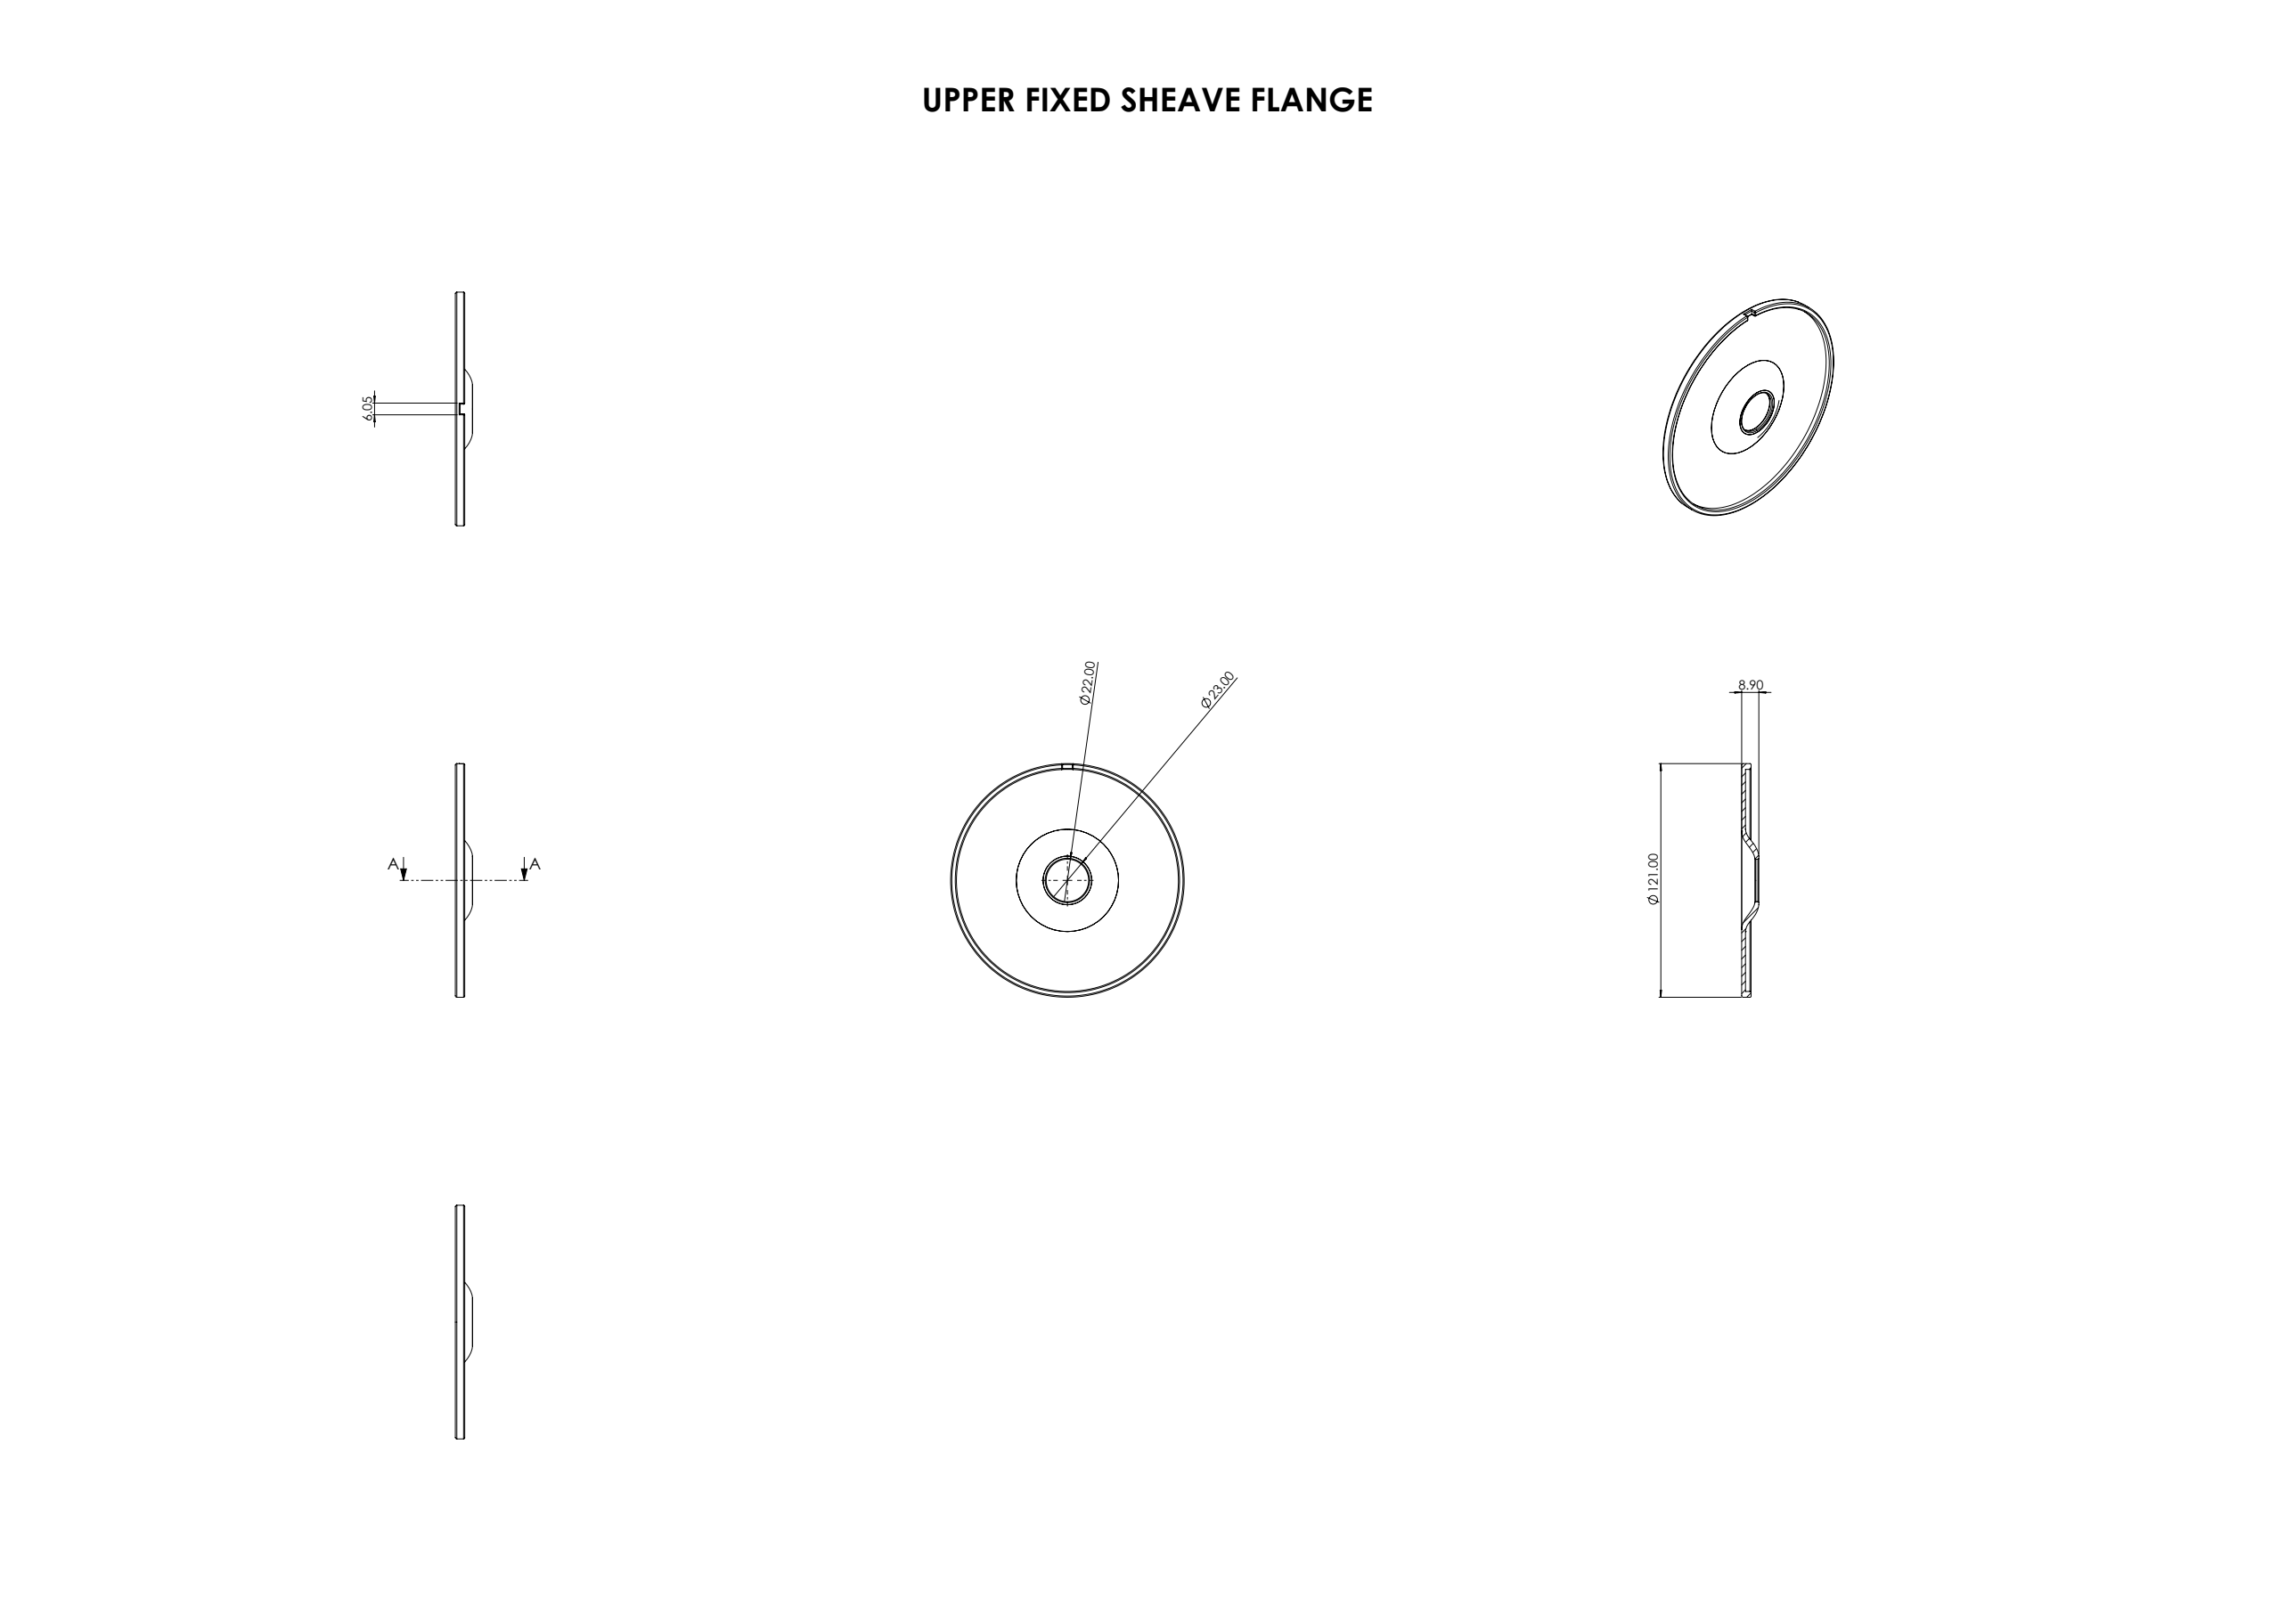
ISO-10303-21;
HEADER;
/* Generated by software containing ST-Developer
 * from STEP Tools, Inc. (www.steptools.com) 
 */

FILE_DESCRIPTION(
/* description */ (''),
/* implementation_level */ '2;1');

FILE_NAME(
/* name */ '01_Upper_Fixed_Sheave_Flange.step',
/* time_stamp */ '2026-10-24T13:41:11-07:00',
/* author */ (''),
/* organization */ (''),
/* preprocessor_version */ 'ST-DEVELOPER v20.2',
/* originating_system */ 'Autodesk Translation Framework v15.15.0.0',
/* authorisation */ '');

FILE_SCHEMA (('AUTOMOTIVE_DESIGN { 1 0 10303 214 3 1 1 }'));
ENDSEC;

DATA;
#10=MECHANICAL_DESIGN_GEOMETRIC_PRESENTATION_REPRESENTATION('',(#121),#12813);
#101=SHAPE_REPRESENTATION_RELATIONSHIP('SRR','None',#12854,#111);
#111=ADVANCED_BREP_SHAPE_REPRESENTATION('',(#131),#12803);
#121=STYLED_ITEM('',(#12960),#131);
#131=MANIFOLD_SOLID_BREP('Body1',#4384);
#141=FACE_BOUND('',#599,.T.);
#142=FACE_BOUND('',#604,.T.);
#143=FACE_BOUND('',#607,.T.);
#169=PLANE('',#4514);
#170=PLANE('',#4517);
#171=PLANE('',#4521);
#172=PLANE('',#4531);
#173=PLANE('',#4540);
#174=PLANE('',#4544);
#175=PLANE('',#4551);
#258=TOROIDAL_SURFACE('',#4511,11.5,0.5);
#259=TOROIDAL_SURFACE('',#4541,60.,0.5);
#260=TOROIDAL_SURFACE('',#4546,58.,0.5);
#261=TOROIDAL_SURFACE('',#4549,58.1,0.6);
#262=TOROIDAL_SURFACE('',#4558,59.9,0.6);
#263=TOROIDAL_SURFACE('',#4559,59.7,0.8);
#290=(
BOUNDED_CURVE()
B_SPLINE_CURVE(5,(#6647,#6648,#6649,#6650,#6651,#6652,#6653,#6654,#6655,
#6656,#6657,#6658,#6659,#6660,#6661,#6662,#6663,#6664,#6665,#6666,#6667,
#6668,#6669,#6670,#6671,#6672,#6673,#6674,#6675,#6676),.UNSPECIFIED.,.F.,
 .F.)
B_SPLINE_CURVE_WITH_KNOTS((6,1,1,1,1,1,1,1,1,1,1,1,1,1,1,1,1,1,1,1,1,1,
1,1,1,6),(8.37815962158244E-5,0.04,0.08,0.12,0.16,0.2,0.24,0.28,0.32,0.36,
0.4,0.44,0.48,0.52,0.56,0.6,0.64,0.68,0.72,0.76,0.8,0.84,0.88,0.92,0.96,
0.969915757295795),.UNSPECIFIED.)
CURVE()
GEOMETRIC_REPRESENTATION_ITEM()
RATIONAL_B_SPLINE_CURVE((1.,1.,1.,1.,1.,1.,1.,1.,1.,1.,1.,1.,1.,1.,1.,1.,
1.,1.,1.,1.,1.,1.,1.,1.,1.,1.,1.,1.,1.,1.))
REPRESENTATION_ITEM('')
);
#291=(
BOUNDED_CURVE()
B_SPLINE_CURVE(5,(#7077,#7078,#7079,#7080,#7081,#7082,#7083,#7084,#7085,
#7086,#7087,#7088,#7089,#7090,#7091,#7092,#7093,#7094,#7095,#7096,#7097,
#7098,#7099,#7100,#7101,#7102,#7103,#7104,#7105,#7106),.UNSPECIFIED.,.F.,
 .F.)
B_SPLINE_CURVE_WITH_KNOTS((6,1,1,1,1,1,1,1,1,1,1,1,1,1,1,1,1,1,1,1,1,1,
1,1,1,6),(0.00142562377953934,0.04,0.08,0.12,0.16,0.2,0.24,0.28,0.32,0.36,
0.4,0.44,0.48,0.52,0.56,0.6,0.64,0.68,0.72,0.76,0.8,0.84,0.88,0.92,0.96,
0.999682925140619),.UNSPECIFIED.)
CURVE()
GEOMETRIC_REPRESENTATION_ITEM()
RATIONAL_B_SPLINE_CURVE((1.,1.,1.,1.,1.,1.,1.,1.,1.,1.,1.,1.,1.,1.,1.,1.,
1.,1.,1.,1.,1.,1.,1.,1.,1.,1.,1.,1.,1.,1.))
REPRESENTATION_ITEM('')
);
#294=(
BOUNDED_SURFACE()
B_SPLINE_SURFACE(5,2,((#6376,#6377,#6378,#6379,#6380,#6381,#6382,#6383,
#6384),(#6385,#6386,#6387,#6388,#6389,#6390,#6391,#6392,#6393),(#6394,#6395,
#6396,#6397,#6398,#6399,#6400,#6401,#6402),(#6403,#6404,#6405,#6406,#6407,
#6408,#6409,#6410,#6411),(#6412,#6413,#6414,#6415,#6416,#6417,#6418,#6419,
#6420),(#6421,#6422,#6423,#6424,#6425,#6426,#6427,#6428,#6429),(#6430,#6431,
#6432,#6433,#6434,#6435,#6436,#6437,#6438),(#6439,#6440,#6441,#6442,#6443,
#6444,#6445,#6446,#6447),(#6448,#6449,#6450,#6451,#6452,#6453,#6454,#6455,
#6456),(#6457,#6458,#6459,#6460,#6461,#6462,#6463,#6464,#6465),(#6466,#6467,
#6468,#6469,#6470,#6471,#6472,#6473,#6474),(#6475,#6476,#6477,#6478,#6479,
#6480,#6481,#6482,#6483),(#6484,#6485,#6486,#6487,#6488,#6489,#6490,#6491,
#6492),(#6493,#6494,#6495,#6496,#6497,#6498,#6499,#6500,#6501),(#6502,#6503,
#6504,#6505,#6506,#6507,#6508,#6509,#6510),(#6511,#6512,#6513,#6514,#6515,
#6516,#6517,#6518,#6519),(#6520,#6521,#6522,#6523,#6524,#6525,#6526,#6527,
#6528),(#6529,#6530,#6531,#6532,#6533,#6534,#6535,#6536,#6537),(#6538,#6539,
#6540,#6541,#6542,#6543,#6544,#6545,#6546),(#6547,#6548,#6549,#6550,#6551,
#6552,#6553,#6554,#6555),(#6556,#6557,#6558,#6559,#6560,#6561,#6562,#6563,
#6564),(#6565,#6566,#6567,#6568,#6569,#6570,#6571,#6572,#6573),(#6574,#6575,
#6576,#6577,#6578,#6579,#6580,#6581,#6582),(#6583,#6584,#6585,#6586,#6587,
#6588,#6589,#6590,#6591),(#6592,#6593,#6594,#6595,#6596,#6597,#6598,#6599,
#6600),(#6601,#6602,#6603,#6604,#6605,#6606,#6607,#6608,#6609),(#6610,#6611,
#6612,#6613,#6614,#6615,#6616,#6617,#6618),(#6619,#6620,#6621,#6622,#6623,
#6624,#6625,#6626,#6627),(#6628,#6629,#6630,#6631,#6632,#6633,#6634,#6635,
#6636),(#6637,#6638,#6639,#6640,#6641,#6642,#6643,#6644,#6645)),
 .UNSPECIFIED.,.F.,.T.,.F.)
B_SPLINE_SURFACE_WITH_KNOTS((6,1,1,1,1,1,1,1,1,1,1,1,1,1,1,1,1,1,1,1,1,
1,1,1,1,6),(3,2,2,2,3),(0.,0.04,0.08,0.12,0.16,0.2,0.24,0.28,0.32,0.36,
0.4,0.44,0.48,0.52,0.56,0.6,0.64,0.68,0.72,0.76,0.8,0.84,0.88,0.92,0.96,
1.),(0.,1.5707963267949,3.14159265358979,4.71238898038469,6.28318530717959),
 .UNSPECIFIED.)
GEOMETRIC_REPRESENTATION_ITEM()
RATIONAL_B_SPLINE_SURFACE(((1.,0.707106781186548,1.,0.707106781186548,1.,
0.707106781186548,1.,0.707106781186548,1.),(1.,0.707106781186548,1.,0.707106781186548,
1.,0.707106781186548,1.,0.707106781186548,1.),(1.,0.707106781186548,1.,
0.707106781186548,1.,0.707106781186548,1.,0.707106781186548,1.),(1.,0.707106781186548,
1.,0.707106781186548,1.,0.707106781186548,1.,0.707106781186548,1.),(1.,
0.707106781186548,1.,0.707106781186548,1.,0.707106781186548,1.,0.707106781186548,
1.),(1.,0.707106781186548,1.,0.707106781186548,1.,0.707106781186548,1.,
0.707106781186548,1.),(1.,0.707106781186548,1.,0.707106781186548,1.,0.707106781186548,
1.,0.707106781186548,1.),(1.,0.707106781186548,1.,0.707106781186548,1.,
0.707106781186548,1.,0.707106781186548,1.),(1.,0.707106781186548,1.,0.707106781186548,
1.,0.707106781186548,1.,0.707106781186548,1.),(1.,0.707106781186548,1.,
0.707106781186548,1.,0.707106781186548,1.,0.707106781186548,1.),(1.,0.707106781186548,
1.,0.707106781186548,1.,0.707106781186548,1.,0.707106781186548,1.),(1.,
0.707106781186548,1.,0.707106781186548,1.,0.707106781186548,1.,0.707106781186548,
1.),(1.,0.707106781186548,1.,0.707106781186548,1.,0.707106781186548,1.,
0.707106781186548,1.),(1.,0.707106781186548,1.,0.707106781186548,1.,0.707106781186548,
1.,0.707106781186548,1.),(1.,0.707106781186548,1.,0.707106781186548,1.,
0.707106781186548,1.,0.707106781186548,1.),(1.,0.707106781186548,1.,0.707106781186548,
1.,0.707106781186548,1.,0.707106781186548,1.),(1.,0.707106781186548,1.,
0.707106781186548,1.,0.707106781186548,1.,0.707106781186548,1.),(1.,0.707106781186548,
1.,0.707106781186548,1.,0.707106781186548,1.,0.707106781186548,1.),(1.,
0.707106781186548,1.,0.707106781186548,1.,0.707106781186548,1.,0.707106781186548,
1.),(1.,0.707106781186548,1.,0.707106781186548,1.,0.707106781186548,1.,
0.707106781186548,1.),(1.,0.707106781186548,1.,0.707106781186548,1.,0.707106781186548,
1.,0.707106781186548,1.),(1.,0.707106781186548,1.,0.707106781186548,1.,
0.707106781186548,1.,0.707106781186548,1.),(1.,0.707106781186548,1.,0.707106781186548,
1.,0.707106781186548,1.,0.707106781186548,1.),(1.,0.707106781186548,1.,
0.707106781186548,1.,0.707106781186548,1.,0.707106781186548,1.),(1.,0.707106781186548,
1.,0.707106781186548,1.,0.707106781186548,1.,0.707106781186548,1.),(1.,
0.707106781186548,1.,0.707106781186548,1.,0.707106781186548,1.,0.707106781186548,
1.),(1.,0.707106781186548,1.,0.707106781186548,1.,0.707106781186548,1.,
0.707106781186548,1.),(1.,0.707106781186548,1.,0.707106781186548,1.,0.707106781186548,
1.,0.707106781186548,1.),(1.,0.707106781186548,1.,0.707106781186548,1.,
0.707106781186548,1.,0.707106781186548,1.),(1.,0.707106781186548,1.,0.707106781186548,
1.,0.707106781186548,1.,0.707106781186548,1.)))
REPRESENTATION_ITEM('')
SURFACE()
);
#295=(
BOUNDED_SURFACE()
B_SPLINE_SURFACE(5,2,((#6806,#6807,#6808,#6809,#6810,#6811,#6812,#6813,
#6814),(#6815,#6816,#6817,#6818,#6819,#6820,#6821,#6822,#6823),(#6824,#6825,
#6826,#6827,#6828,#6829,#6830,#6831,#6832),(#6833,#6834,#6835,#6836,#6837,
#6838,#6839,#6840,#6841),(#6842,#6843,#6844,#6845,#6846,#6847,#6848,#6849,
#6850),(#6851,#6852,#6853,#6854,#6855,#6856,#6857,#6858,#6859),(#6860,#6861,
#6862,#6863,#6864,#6865,#6866,#6867,#6868),(#6869,#6870,#6871,#6872,#6873,
#6874,#6875,#6876,#6877),(#6878,#6879,#6880,#6881,#6882,#6883,#6884,#6885,
#6886),(#6887,#6888,#6889,#6890,#6891,#6892,#6893,#6894,#6895),(#6896,#6897,
#6898,#6899,#6900,#6901,#6902,#6903,#6904),(#6905,#6906,#6907,#6908,#6909,
#6910,#6911,#6912,#6913),(#6914,#6915,#6916,#6917,#6918,#6919,#6920,#6921,
#6922),(#6923,#6924,#6925,#6926,#6927,#6928,#6929,#6930,#6931),(#6932,#6933,
#6934,#6935,#6936,#6937,#6938,#6939,#6940),(#6941,#6942,#6943,#6944,#6945,
#6946,#6947,#6948,#6949),(#6950,#6951,#6952,#6953,#6954,#6955,#6956,#6957,
#6958),(#6959,#6960,#6961,#6962,#6963,#6964,#6965,#6966,#6967),(#6968,#6969,
#6970,#6971,#6972,#6973,#6974,#6975,#6976),(#6977,#6978,#6979,#6980,#6981,
#6982,#6983,#6984,#6985),(#6986,#6987,#6988,#6989,#6990,#6991,#6992,#6993,
#6994),(#6995,#6996,#6997,#6998,#6999,#7000,#7001,#7002,#7003),(#7004,#7005,
#7006,#7007,#7008,#7009,#7010,#7011,#7012),(#7013,#7014,#7015,#7016,#7017,
#7018,#7019,#7020,#7021),(#7022,#7023,#7024,#7025,#7026,#7027,#7028,#7029,
#7030),(#7031,#7032,#7033,#7034,#7035,#7036,#7037,#7038,#7039),(#7040,#7041,
#7042,#7043,#7044,#7045,#7046,#7047,#7048),(#7049,#7050,#7051,#7052,#7053,
#7054,#7055,#7056,#7057),(#7058,#7059,#7060,#7061,#7062,#7063,#7064,#7065,
#7066),(#7067,#7068,#7069,#7070,#7071,#7072,#7073,#7074,#7075)),
 .UNSPECIFIED.,.F.,.T.,.F.)
B_SPLINE_SURFACE_WITH_KNOTS((6,1,1,1,1,1,1,1,1,1,1,1,1,1,1,1,1,1,1,1,1,
1,1,1,1,6),(3,2,2,2,3),(0.,0.04,0.08,0.12,0.16,0.2,0.24,0.28,0.32,0.36,
0.4,0.44,0.48,0.52,0.56,0.6,0.64,0.68,0.72,0.76,0.8,0.84,0.88,0.92,0.96,
1.),(0.,1.5707963267949,3.14159265358979,4.71238898038469,6.28318530717959),
 .UNSPECIFIED.)
GEOMETRIC_REPRESENTATION_ITEM()
RATIONAL_B_SPLINE_SURFACE(((1.,0.707106781186548,1.,0.707106781186548,1.,
0.707106781186548,1.,0.707106781186548,1.),(1.,0.707106781186548,1.,0.707106781186548,
1.,0.707106781186548,1.,0.707106781186548,1.),(1.,0.707106781186548,1.,
0.707106781186548,1.,0.707106781186548,1.,0.707106781186548,1.),(1.,0.707106781186548,
1.,0.707106781186548,1.,0.707106781186548,1.,0.707106781186548,1.),(1.,
0.707106781186548,1.,0.707106781186548,1.,0.707106781186548,1.,0.707106781186548,
1.),(1.,0.707106781186548,1.,0.707106781186548,1.,0.707106781186548,1.,
0.707106781186548,1.),(1.,0.707106781186548,1.,0.707106781186548,1.,0.707106781186548,
1.,0.707106781186548,1.),(1.,0.707106781186548,1.,0.707106781186548,1.,
0.707106781186548,1.,0.707106781186548,1.),(1.,0.707106781186548,1.,0.707106781186548,
1.,0.707106781186548,1.,0.707106781186548,1.),(1.,0.707106781186548,1.,
0.707106781186548,1.,0.707106781186548,1.,0.707106781186548,1.),(1.,0.707106781186548,
1.,0.707106781186548,1.,0.707106781186548,1.,0.707106781186548,1.),(1.,
0.707106781186548,1.,0.707106781186548,1.,0.707106781186548,1.,0.707106781186548,
1.),(1.,0.707106781186548,1.,0.707106781186548,1.,0.707106781186548,1.,
0.707106781186548,1.),(1.,0.707106781186548,1.,0.707106781186548,1.,0.707106781186548,
1.,0.707106781186548,1.),(1.,0.707106781186548,1.,0.707106781186548,1.,
0.707106781186548,1.,0.707106781186548,1.),(1.,0.707106781186548,1.,0.707106781186548,
1.,0.707106781186548,1.,0.707106781186548,1.),(1.,0.707106781186548,1.,
0.707106781186548,1.,0.707106781186548,1.,0.707106781186548,1.),(1.,0.707106781186548,
1.,0.707106781186548,1.,0.707106781186548,1.,0.707106781186548,1.),(1.,
0.707106781186548,1.,0.707106781186548,1.,0.707106781186548,1.,0.707106781186548,
1.),(1.,0.707106781186548,1.,0.707106781186548,1.,0.707106781186548,1.,
0.707106781186548,1.),(1.,0.707106781186548,1.,0.707106781186548,1.,0.707106781186548,
1.,0.707106781186548,1.),(1.,0.707106781186548,1.,0.707106781186548,1.,
0.707106781186548,1.,0.707106781186548,1.),(1.,0.707106781186548,1.,0.707106781186548,
1.,0.707106781186548,1.,0.707106781186548,1.),(1.,0.707106781186548,1.,
0.707106781186548,1.,0.707106781186548,1.,0.707106781186548,1.),(1.,0.707106781186548,
1.,0.707106781186548,1.,0.707106781186548,1.,0.707106781186548,1.),(1.,
0.707106781186548,1.,0.707106781186548,1.,0.707106781186548,1.,0.707106781186548,
1.),(1.,0.707106781186548,1.,0.707106781186548,1.,0.707106781186548,1.,
0.707106781186548,1.),(1.,0.707106781186548,1.,0.707106781186548,1.,0.707106781186548,
1.,0.707106781186548,1.),(1.,0.707106781186548,1.,0.707106781186548,1.,
0.707106781186548,1.,0.707106781186548,1.),(1.,0.707106781186548,1.,0.707106781186548,
1.,0.707106781186548,1.,0.707106781186548,1.)))
REPRESENTATION_ITEM('')
SURFACE()
);
#298=B_SPLINE_SURFACE_WITH_KNOTS('',3,3,((#6289,#6290,#6291,#6292,#6293,
#6294,#6295,#6296,#6297,#6298,#6299,#6300,#6301,#6302,#6303,#6304,#6305),
(#6306,#6307,#6308,#6309,#6310,#6311,#6312,#6313,#6314,#6315,#6316,#6317,
#6318,#6319,#6320,#6321,#6322),(#6323,#6324,#6325,#6326,#6327,#6328,#6329,
#6330,#6331,#6332,#6333,#6334,#6335,#6336,#6337,#6338,#6339),(#6340,#6341,
#6342,#6343,#6344,#6345,#6346,#6347,#6348,#6349,#6350,#6351,#6352,#6353,
#6354,#6355,#6356)),.UNSPECIFIED.,.F.,.T.,.F.,(4,4),(4,1,1,1,1,1,1,1,1,
1,1,1,1,1,4),(0.316273000492814,1.),(1.5707963267949,2.01959527730772,2.46839422782055,
2.91719317833338,3.36599212884621,3.96439072952998,4.26359002987186,4.56278933021375,
5.16118793089752,5.4603872312394,6.05878583192317,6.35798513226506,6.95638373294883,
7.40518268346166,7.85398163397448),.UNSPECIFIED.);
#299=B_SPLINE_SURFACE_WITH_KNOTS('',3,3,((#6719,#6720,#6721,#6722,#6723,
#6724,#6725,#6726,#6727,#6728,#6729,#6730,#6731,#6732,#6733,#6734,#6735),
(#6736,#6737,#6738,#6739,#6740,#6741,#6742,#6743,#6744,#6745,#6746,#6747,
#6748,#6749,#6750,#6751,#6752),(#6753,#6754,#6755,#6756,#6757,#6758,#6759,
#6760,#6761,#6762,#6763,#6764,#6765,#6766,#6767,#6768,#6769),(#6770,#6771,
#6772,#6773,#6774,#6775,#6776,#6777,#6778,#6779,#6780,#6781,#6782,#6783,
#6784,#6785,#6786)),.UNSPECIFIED.,.F.,.T.,.F.,(4,4),(4,1,1,1,1,1,1,1,1,
1,1,1,1,1,4),(0.,1.),(1.5707963267949,2.01959527730772,2.46839422782055,
2.91719317833338,3.36599212884621,3.66519142918809,4.26359002987186,4.56278933021375,
5.16118793089752,5.4603872312394,6.05878583192317,6.35798513226506,6.95638373294883,
7.40518268346166,7.85398163397448),.UNSPECIFIED.);
#300=B_SPLINE_SURFACE_WITH_KNOTS('',3,3,((#7126,#7127,#7128,#7129,#7130,
#7131,#7132,#7133,#7134,#7135,#7136,#7137,#7138,#7139,#7140,#7141,#7142,
#7143,#7144),(#7145,#7146,#7147,#7148,#7149,#7150,#7151,#7152,#7153,#7154,
#7155,#7156,#7157,#7158,#7159,#7160,#7161,#7162,#7163),(#7164,#7165,#7166,
#7167,#7168,#7169,#7170,#7171,#7172,#7173,#7174,#7175,#7176,#7177,#7178,
#7179,#7180,#7181,#7182),(#7183,#7184,#7185,#7186,#7187,#7188,#7189,#7190,
#7191,#7192,#7193,#7194,#7195,#7196,#7197,#7198,#7199,#7200,#7201)),
 .UNSPECIFIED.,.F.,.T.,.F.,(4,4),(4,1,1,1,1,1,1,1,1,1,1,1,1,1,1,1,4),(0.,
1.),(1.5707963267949,2.01959527730772,2.46839422782055,2.91719317833338,
3.36599212884621,3.66519142918809,3.96439072952998,4.26359002987186,4.56278933021375,
5.16118793089752,5.4603872312394,5.75958653158129,6.05878583192317,6.35798513226506,
6.95638373294883,7.40518268346166,7.85398163397448),.UNSPECIFIED.);
#301=B_SPLINE_SURFACE_WITH_KNOTS('',3,3,((#7228,#7229,#7230,#7231,#7232,
#7233,#7234,#7235,#7236,#7237,#7238,#7239,#7240,#7241,#7242,#7243,#7244,
#7245,#7246),(#7247,#7248,#7249,#7250,#7251,#7252,#7253,#7254,#7255,#7256,
#7257,#7258,#7259,#7260,#7261,#7262,#7263,#7264,#7265),(#7266,#7267,#7268,
#7269,#7270,#7271,#7272,#7273,#7274,#7275,#7276,#7277,#7278,#7279,#7280,
#7281,#7282,#7283,#7284),(#7285,#7286,#7287,#7288,#7289,#7290,#7291,#7292,
#7293,#7294,#7295,#7296,#7297,#7298,#7299,#7300,#7301,#7302,#7303)),
 .UNSPECIFIED.,.F.,.T.,.F.,(4,4),(4,1,1,1,1,1,1,1,1,1,1,1,1,1,1,1,4),(0.,
1.),(1.5707963267949,2.01959527730772,2.46839422782055,2.91719317833338,
3.36599212884621,3.66519142918809,3.96439072952998,4.26359002987186,4.56278933021375,
5.16118793089752,5.4603872312394,5.75958653158129,6.05878583192317,6.35798513226506,
6.95638373294883,7.40518268346166,7.85398163397448),.UNSPECIFIED.);
#302=B_SPLINE_SURFACE_WITH_KNOTS('',3,3,((#7382,#7383,#7384,#7385,#7386),
(#7387,#7388,#7389,#7390,#7391),(#7392,#7393,#7394,#7395,#7396),(#7397,
#7398,#7399,#7400,#7401),(#7402,#7403,#7404,#7405,#7406)),.UNSPECIFIED.,
 .F.,.F.,.F.,(4,1,4),(4,1,4),(0.,0.5,1.),(0.,0.00785862436681818,0.0157172487336364),
 .UNSPECIFIED.);
#303=B_SPLINE_SURFACE_WITH_KNOTS('',3,3,((#7426,#7427,#7428,#7429,#7430),
(#7431,#7432,#7433,#7434,#7435),(#7436,#7437,#7438,#7439,#7440),(#7441,
#7442,#7443,#7444,#7445),(#7446,#7447,#7448,#7449,#7450)),.UNSPECIFIED.,
 .F.,.F.,.F.,(4,1,4),(4,1,4),(0.,0.5,1.),(0.,0.00785894990202256,0.0157178998040451),
 .UNSPECIFIED.);
#304=B_SPLINE_SURFACE_WITH_KNOTS('',3,3,((#7510,#7511,#7512,#7513,#7514),
(#7515,#7516,#7517,#7518,#7519),(#7520,#7521,#7522,#7523,#7524),(#7525,
#7526,#7527,#7528,#7529),(#7530,#7531,#7532,#7533,#7534)),.UNSPECIFIED.,
 .F.,.F.,.F.,(4,1,4),(4,1,4),(0.,0.5,1.),(1.02053899928999E-18,0.00785895027235015,
0.0157179005447003),.UNSPECIFIED.);
#305=B_SPLINE_SURFACE_WITH_KNOTS('',3,3,((#7554,#7555,#7556,#7557,#7558),
(#7559,#7560,#7561,#7562,#7563),(#7564,#7565,#7566,#7567,#7568),(#7569,
#7570,#7571,#7572,#7573),(#7574,#7575,#7576,#7577,#7578)),.UNSPECIFIED.,
 .F.,.F.,.F.,(4,1,4),(4,1,4),(0.,0.5,1.),(0.,0.00785862401697905,0.0157172480339581),
 .UNSPECIFIED.);
#324=FACE_OUTER_BOUND('',#594,.T.);
#325=FACE_OUTER_BOUND('',#595,.T.);
#326=FACE_OUTER_BOUND('',#596,.T.);
#327=FACE_OUTER_BOUND('',#597,.T.);
#328=FACE_OUTER_BOUND('',#598,.T.);
#329=FACE_OUTER_BOUND('',#600,.T.);
#330=FACE_OUTER_BOUND('',#601,.T.);
#331=FACE_OUTER_BOUND('',#602,.T.);
#332=FACE_OUTER_BOUND('',#603,.T.);
#333=FACE_OUTER_BOUND('',#605,.T.);
#334=FACE_OUTER_BOUND('',#606,.T.);
#335=FACE_OUTER_BOUND('',#608,.T.);
#336=FACE_OUTER_BOUND('',#609,.T.);
#337=FACE_OUTER_BOUND('',#610,.T.);
#338=FACE_OUTER_BOUND('',#611,.T.);
#339=FACE_OUTER_BOUND('',#612,.T.);
#340=FACE_OUTER_BOUND('',#613,.T.);
#341=FACE_OUTER_BOUND('',#614,.T.);
#342=FACE_OUTER_BOUND('',#615,.T.);
#343=FACE_OUTER_BOUND('',#616,.T.);
#344=FACE_OUTER_BOUND('',#617,.T.);
#345=FACE_OUTER_BOUND('',#618,.T.);
#346=FACE_OUTER_BOUND('',#619,.T.);
#347=FACE_OUTER_BOUND('',#620,.T.);
#348=FACE_OUTER_BOUND('',#621,.T.);
#349=FACE_OUTER_BOUND('',#622,.T.);
#350=FACE_OUTER_BOUND('',#623,.T.);
#351=FACE_OUTER_BOUND('',#624,.T.);
#352=FACE_OUTER_BOUND('',#625,.T.);
#353=FACE_OUTER_BOUND('',#626,.T.);
#354=FACE_OUTER_BOUND('',#627,.T.);
#355=FACE_OUTER_BOUND('',#628,.T.);
#594=EDGE_LOOP('',(#2767,#2768,#2769,#2770,#2771,#2772));
#595=EDGE_LOOP('',(#2773,#2774,#2775,#2776,#2777));
#596=EDGE_LOOP('',(#2778,#2779,#2780,#2781));
#597=EDGE_LOOP('',(#2782,#2783,#2784,#2785,#2786));
#598=EDGE_LOOP('',(#2787));
#599=EDGE_LOOP('',(#2788));
#600=EDGE_LOOP('',(#2789,#2790,#2791,#2792));
#601=EDGE_LOOP('',(#2793,#2794,#2795,#2796));
#602=EDGE_LOOP('',(#2797,#2798,#2799,#2800));
#603=EDGE_LOOP('',(#2801,#2802));
#604=EDGE_LOOP('',(#2803));
#605=EDGE_LOOP('',(#2804,#2805,#2806,#2807));
#606=EDGE_LOOP('',(#2808));
#607=EDGE_LOOP('',(#2809));
#608=EDGE_LOOP('',(#2810,#2811,#2812,#2813,#2814));
#609=EDGE_LOOP('',(#2815,#2816,#2817,#2818));
#610=EDGE_LOOP('',(#2819,#2820,#2821,#2822));
#611=EDGE_LOOP('',(#2823,#2824,#2825,#2826));
#612=EDGE_LOOP('',(#2827,#2828,#2829,#2830));
#613=EDGE_LOOP('',(#2831,#2832,#2833,#2834,#2835,#2836,#2837));
#614=EDGE_LOOP('',(#2838,#2839,#2840,#2841));
#615=EDGE_LOOP('',(#2842,#2843,#2844,#2845));
#616=EDGE_LOOP('',(#2846,#2847,#2848,#2849));
#617=EDGE_LOOP('',(#2850,#2851,#2852,#2853));
#618=EDGE_LOOP('',(#2854,#2855,#2856,#2857,#2858));
#619=EDGE_LOOP('',(#2859,#2860,#2861,#2862,#2863,#2864,#2865));
#620=EDGE_LOOP('',(#2866,#2867,#2868,#2869));
#621=EDGE_LOOP('',(#2870,#2871,#2872,#2873,#2874,#2875));
#622=EDGE_LOOP('',(#2876,#2877,#2878,#2879,#2880,#2881));
#623=EDGE_LOOP('',(#2882,#2883,#2884,#2885));
#624=EDGE_LOOP('',(#2886,#2887,#2888,#2889));
#625=EDGE_LOOP('',(#2890,#2891,#2892,#2893));
#626=EDGE_LOOP('',(#2894,#2895,#2896,#2897,#2898,#2899,#2900,#2901,#2902));
#627=EDGE_LOOP('',(#2903,#2904,#2905,#2906,#2907));
#628=EDGE_LOOP('',(#2908,#2909,#2910,#2911,#2912));
#892=CIRCLE('',#4508,11.05);
#893=CIRCLE('',#4509,11.05);
#894=CIRCLE('',#4510,0.499999999999999);
#895=CIRCLE('',#4512,0.5);
#896=CIRCLE('',#4513,11.5);
#897=CIRCLE('',#4515,0.500000000000007);
#898=CIRCLE('',#4516,0.499999999999999);
#899=CIRCLE('',#4518,57.5);
#900=CIRCLE('',#4519,57.5);
#901=CIRCLE('',#4520,0.499999999999989);
#902=CIRCLE('',#4522,59.7);
#903=CIRCLE('',#4524,0.5);
#904=CIRCLE('',#4525,0.5);
#905=CIRCLE('',#4526,0.5);
#906=CIRCLE('',#4528,0.5);
#907=CIRCLE('',#4529,0.5);
#908=CIRCLE('',#4533,0.5);
#909=CIRCLE('',#4534,0.5);
#910=CIRCLE('',#4536,0.5);
#911=CIRCLE('',#4537,0.5);
#912=CIRCLE('',#4539,0.5);
#913=CIRCLE('',#4542,60.);
#914=CIRCLE('',#4543,60.5);
#915=CIRCLE('',#4545,58.);
#916=CIRCLE('',#4548,57.5);
#917=CIRCLE('',#4550,58.1);
#918=CIRCLE('',#4552,59.9);
#919=CIRCLE('',#4554,60.5);
#920=CIRCLE('',#4555,60.5);
#921=CIRCLE('',#4556,60.5);
#922=CIRCLE('',#4557,60.5);
#923=CIRCLE('',#4560,0.8);
#1123=LINE('',#6285,#1353);
#1124=LINE('',#7363,#1354);
#1125=LINE('',#7367,#1355);
#1126=LINE('',#7424,#1356);
#1127=LINE('',#7425,#1357);
#1128=LINE('',#7480,#1358);
#1129=LINE('',#7481,#1359);
#1130=LINE('',#7484,#1360);
#1131=LINE('',#7506,#1361);
#1132=LINE('',#7509,#1362);
#1133=LINE('',#7552,#1363);
#1134=LINE('',#7553,#1364);
#1135=LINE('',#7609,#1365);
#1136=LINE('',#7611,#1366);
#1137=LINE('',#7619,#1367);
#1138=LINE('',#7636,#1368);
#1353=VECTOR('',#5010,11.05);
#1354=VECTOR('',#5045,10.);
#1355=VECTOR('',#5048,10.);
#1356=VECTOR('',#5055,10.);
#1357=VECTOR('',#5056,10.);
#1358=VECTOR('',#5061,10.);
#1359=VECTOR('',#5062,10.);
#1360=VECTOR('',#5065,10.);
#1361=VECTOR('',#5068,10.);
#1362=VECTOR('',#5071,10.);
#1363=VECTOR('',#5078,10.);
#1364=VECTOR('',#5079,10.);
#1365=VECTOR('',#5084,10.);
#1366=VECTOR('',#5085,10.);
#1367=VECTOR('',#5090,10.);
#1368=VECTOR('',#5119,60.5);
#1583=B_SPLINE_CURVE_WITH_KNOTS('',3,(#6237,#6238,#6239,#6240,#6241,#6242,
#6243,#6244,#6245,#6246,#6247,#6248,#6249,#6250,#6251,#6252,#6253,#6254,
#6255,#6256,#6257,#6258,#6259,#6260,#6261),.UNSPECIFIED.,.F.,.F.,(4,3,3,
3,3,3,3,3,4),(-6.96374017603088,-6.4663927644122,-5.96904535279352,-5.47169794117485,
-4.97435052955617,-4.31122064739794,-3.97965570631882,-3.6480907652397,
-3.48231742770748),.UNSPECIFIED.);
#1584=B_SPLINE_CURVE_WITH_KNOTS('',3,(#6262,#6263,#6264,#6265,#6266,#6267,
#6268,#6269,#6270,#6271,#6272,#6273,#6274,#6275,#6276,#6277,#6278,#6279,
#6280,#6281,#6282,#6283),.UNSPECIFIED.,.F.,.F.,(4,3,3,3,3,3,3,4),(-3.48231742770748,
-2.98483567920087,-2.65318727040077,-1.98989045280058,-1.65824204400048,
-0.994945226400289,-0.497472613200144,0.),.UNSPECIFIED.);
#1585=B_SPLINE_CURVE_WITH_KNOTS('',3,(#6359,#6360,#6361,#6362,#6363,#6364,
#6365,#6366,#6367,#6368,#6369,#6370,#6371,#6372,#6373,#6374,#6375),
 .UNSPECIFIED.,.T.,.F.,(4,1,1,1,1,1,1,1,1,1,1,1,1,1,4),(-7.85398163397448,
-7.40518268346166,-6.95638373294883,-6.35798513226506,-6.05878583192317,
-5.4603872312394,-5.16118793089752,-4.56278933021375,-4.26359002987186,
-3.96439072952998,-3.36599212884621,-2.91719317833338,-2.46839422782055,
-2.01959527730772,-1.5707963267949),.UNSPECIFIED.);
#1586=B_SPLINE_CURVE_WITH_KNOTS('',3,(#6677,#6678,#6679,#6680,#6681,#6682,
#6683,#6684,#6685,#6686,#6687,#6688,#6689,#6690,#6691,#6692,#6693,#6694,
#6695),.UNSPECIFIED.,.T.,.F.,(4,1,1,1,1,1,1,1,1,1,1,1,1,1,1,1,4),(1.5707963267949,
2.01959527730772,2.46839422782055,2.91719317833338,3.36599212884621,3.66519142918809,
3.96439072952998,4.26359002987186,4.56278933021375,5.16118793089752,5.4603872312394,
5.75958653158129,6.05878583192317,6.35798513226506,6.95638373294883,7.40518268346166,
7.85398163397448),.UNSPECIFIED.);
#1587=B_SPLINE_CURVE_WITH_KNOTS('',3,(#6702,#6703,#6704,#6705,#6706,#6707,
#6708,#6709,#6710,#6711,#6712,#6713,#6714,#6715,#6716,#6717,#6718),
 .UNSPECIFIED.,.T.,.F.,(4,1,1,1,1,1,1,1,1,1,1,1,1,1,4),(-7.85398163397448,
-7.40518268346166,-6.95638373294883,-6.35798513226506,-6.05878583192317,
-5.4603872312394,-5.16118793089752,-4.56278933021375,-4.26359002987186,
-3.66519142918809,-3.36599212884621,-2.91719317833338,-2.46839422782055,
-2.01959527730772,-1.5707963267949),.UNSPECIFIED.);
#1588=B_SPLINE_CURVE_WITH_KNOTS('',3,(#6789,#6790,#6791,#6792,#6793,#6794,
#6795,#6796,#6797,#6798,#6799,#6800,#6801,#6802,#6803,#6804,#6805),
 .UNSPECIFIED.,.T.,.F.,(4,1,1,1,1,1,1,1,1,1,1,1,1,1,4),(1.5707963267949,
2.01959527730772,2.46839422782055,2.91719317833338,3.36599212884621,3.66519142918809,
4.26359002987186,4.56278933021375,5.16118793089752,5.4603872312394,6.05878583192317,
6.35798513226506,6.95638373294883,7.40518268346166,7.85398163397448),
 .UNSPECIFIED.);
#1589=B_SPLINE_CURVE_WITH_KNOTS('',3,(#7107,#7108,#7109,#7110,#7111,#7112,
#7113,#7114,#7115,#7116,#7117,#7118,#7119,#7120,#7121,#7122,#7123,#7124,
#7125),.UNSPECIFIED.,.T.,.F.,(4,1,1,1,1,1,1,1,1,1,1,1,1,1,1,1,4),(-7.85398163397448,
-7.40518268346166,-6.95638373294883,-6.35798513226506,-6.05878583192317,
-5.75958653158129,-5.4603872312394,-5.16118793089752,-4.56278933021375,
-4.26359002987186,-3.96439072952998,-3.66519142918809,-3.36599212884621,
-2.91719317833338,-2.46839422782055,-2.01959527730772,-1.5707963267949),
 .UNSPECIFIED.);
#1590=B_SPLINE_CURVE_WITH_KNOTS('',3,(#7204,#7205,#7206,#7207,#7208,#7209,
#7210,#7211,#7212,#7213,#7214,#7215,#7216,#7217,#7218,#7219,#7220,#7221,
#7222),.UNSPECIFIED.,.T.,.F.,(4,1,1,1,1,1,1,1,1,1,1,1,1,1,1,1,4),(1.5707963267949,
2.01959527730772,2.46839422782055,2.91719317833338,3.36599212884621,3.66519142918809,
3.96439072952998,4.26359002987186,4.56278933021375,5.16118793089752,5.4603872312394,
5.75958653158129,6.05878583192317,6.35798513226506,6.95638373294883,7.40518268346166,
7.85398163397448),.UNSPECIFIED.);
#1591=B_SPLINE_CURVE_WITH_KNOTS('',3,(#7306,#7307,#7308,#7309,#7310,#7311,
#7312,#7313,#7314,#7315,#7316,#7317,#7318,#7319,#7320,#7321,#7322,#7323,
#7324,#7325,#7326,#7327,#7328,#7329,#7330,#7331,#7332,#7333,#7334,#7335,
#7336,#7337,#7338,#7339,#7340,#7341,#7342,#7343,#7344,#7345,#7346,#7347,
#7348,#7349,#7350,#7351,#7352,#7353,#7354),.UNSPECIFIED.,.T.,.F.,(4,3,3,
3,3,3,3,3,3,3,3,3,3,3,3,3,4),(-7.85398163397448,-7.40518268346166,-6.95638373294883,
-6.35798513226506,-6.05878583192317,-5.75958653158129,-5.4603872312394,
-5.16118793089752,-4.56278933021375,-4.26359002987186,-3.96439072952998,
-3.66519142918809,-3.36599212884621,-2.91719317833338,-2.46839422782055,
-2.01959527730772,-1.5707963267949),.UNSPECIFIED.);
#1592=B_SPLINE_CURVE_WITH_KNOTS('',3,(#7368,#7369,#7370,#7371,#7372,#7373,
#7374,#7375,#7376,#7377,#7378,#7379,#7380,#7381),.UNSPECIFIED.,.F.,.F.,
(4,2,2,2,2,2,4),(-0.107735848698753,-0.106444261823602,-0.0883469717566643,
-0.066319510943676,-0.0374807627664021,0.,0.000337595117382213),
 .UNSPECIFIED.);
#1593=B_SPLINE_CURVE_WITH_KNOTS('',3,(#7410,#7411,#7412,#7413,#7414),
 .UNSPECIFIED.,.F.,.F.,(4,1,4),(-0.0157172487336364,-0.00785862436681818,
0.),.UNSPECIFIED.);
#1594=B_SPLINE_CURVE_WITH_KNOTS('',3,(#7415,#7416,#7417,#7418,#7419),
 .UNSPECIFIED.,.F.,.F.,(4,1,4),(0.,0.00785862436681818,0.0157172487336364),
 .UNSPECIFIED.);
#1595=B_SPLINE_CURVE_WITH_KNOTS('',3,(#7454,#7455,#7456,#7457,#7458),
 .UNSPECIFIED.,.F.,.F.,(4,1,4),(-0.0157178998040451,-0.00785894990202256,
0.),.UNSPECIFIED.);
#1596=B_SPLINE_CURVE_WITH_KNOTS('',3,(#7459,#7460,#7461,#7462,#7463),
 .UNSPECIFIED.,.F.,.F.,(4,1,4),(0.,0.00785894990202256,0.0157178998040451),
 .UNSPECIFIED.);
#1597=B_SPLINE_CURVE_WITH_KNOTS('',3,(#7466,#7467,#7468,#7469,#7470,#7471,
#7472,#7473,#7474,#7475,#7476,#7477,#7478,#7479),.UNSPECIFIED.,.F.,.F.,
(4,2,2,2,2,2,4),(-0.223861268001062,-0.223443477302026,-0.194339722291654,
-0.164729520611538,-0.141542392329575,-0.123303095351833,-0.110634522469103),
 .UNSPECIFIED.);
#1598=B_SPLINE_CURVE_WITH_KNOTS('',3,(#7485,#7486,#7487,#7488),
 .UNSPECIFIED.,.F.,.F.,(4,4),(0.0740823244647065,0.0764086756743631),
 .UNSPECIFIED.);
#1599=B_SPLINE_CURVE_WITH_KNOTS('',3,(#7491,#7492,#7493,#7494,#7495,#7496,
#7497,#7498,#7499,#7500,#7501,#7502,#7503,#7504),.UNSPECIFIED.,.F.,.F.,
(4,2,2,2,2,2,4),(-0.0929971191805655,-0.0825534377905717,-0.0675173790191802,
-0.0484024414197425,-0.0239924691911123,0.,0.000344417085089716),
 .UNSPECIFIED.);
#1600=B_SPLINE_CURVE_WITH_KNOTS('',3,(#7538,#7539,#7540,#7541,#7542),
 .UNSPECIFIED.,.F.,.F.,(4,1,4),(-0.0157179005447003,-0.00785895027235015,
-1.02053899928999E-18),.UNSPECIFIED.);
#1601=B_SPLINE_CURVE_WITH_KNOTS('',3,(#7543,#7544,#7545,#7546,#7547),
 .UNSPECIFIED.,.F.,.F.,(4,1,4),(1.02053899928999E-18,0.00785895027235015,
0.0157179005447003),.UNSPECIFIED.);
#1602=B_SPLINE_CURVE_WITH_KNOTS('',3,(#7582,#7583,#7584,#7585,#7586),
 .UNSPECIFIED.,.F.,.F.,(4,1,4),(-0.0157172480339581,-0.00785862401697905,
0.),.UNSPECIFIED.);
#1603=B_SPLINE_CURVE_WITH_KNOTS('',3,(#7587,#7588,#7589,#7590,#7591),
 .UNSPECIFIED.,.F.,.F.,(4,1,4),(0.,0.00785862401697905,0.0157172480339581),
 .UNSPECIFIED.);
#1604=B_SPLINE_CURVE_WITH_KNOTS('',3,(#7595,#7596,#7597,#7598,#7599,#7600,
#7601,#7602,#7603,#7604,#7605,#7606,#7607,#7608),.UNSPECIFIED.,.F.,.F.,
(4,2,2,2,2,2,4),(-0.184461049750143,-0.184182901618329,-0.153302110980918,
-0.129541566131588,-0.1113929118506,-0.0964823661623737,-0.0954182142898604),
 .UNSPECIFIED.);
#1605=B_SPLINE_CURVE_WITH_KNOTS('',3,(#7615,#7616,#7617,#7618),
 .UNSPECIFIED.,.F.,.F.,(4,4),(0.21992163243666,0.222247983646316),
 .UNSPECIFIED.);
#1745=VERTEX_POINT('',#6235);
#1746=VERTEX_POINT('',#6236);
#1747=VERTEX_POINT('',#6284);
#1748=VERTEX_POINT('',#6286);
#1749=VERTEX_POINT('',#6357);
#1750=VERTEX_POINT('',#6646);
#1751=VERTEX_POINT('',#6697);
#1752=VERTEX_POINT('',#6701);
#1753=VERTEX_POINT('',#6787);
#1754=VERTEX_POINT('',#7076);
#1755=VERTEX_POINT('',#7202);
#1756=VERTEX_POINT('',#7224);
#1757=VERTEX_POINT('',#7225);
#1758=VERTEX_POINT('',#7304);
#1759=VERTEX_POINT('',#7356);
#1760=VERTEX_POINT('',#7359);
#1761=VERTEX_POINT('',#7360);
#1762=VERTEX_POINT('',#7362);
#1763=VERTEX_POINT('',#7364);
#1764=VERTEX_POINT('',#7366);
#1765=VERTEX_POINT('',#7407);
#1766=VERTEX_POINT('',#7408);
#1767=VERTEX_POINT('',#7421);
#1768=VERTEX_POINT('',#7422);
#1769=VERTEX_POINT('',#7451);
#1770=VERTEX_POINT('',#7452);
#1771=VERTEX_POINT('',#7465);
#1772=VERTEX_POINT('',#7483);
#1773=VERTEX_POINT('',#7490);
#1774=VERTEX_POINT('',#7505);
#1775=VERTEX_POINT('',#7507);
#1776=VERTEX_POINT('',#7535);
#1777=VERTEX_POINT('',#7536);
#1778=VERTEX_POINT('',#7549);
#1779=VERTEX_POINT('',#7550);
#1780=VERTEX_POINT('',#7579);
#1781=VERTEX_POINT('',#7580);
#1782=VERTEX_POINT('',#7593);
#1783=VERTEX_POINT('',#7594);
#1784=VERTEX_POINT('',#7610);
#1785=VERTEX_POINT('',#7614);
#1786=VERTEX_POINT('',#7633);
#1787=VERTEX_POINT('',#7635);
#1788=VERTEX_POINT('',#7637);
#2136=EDGE_CURVE('',#1745,#1746,#1583,.T.);
#2137=EDGE_CURVE('',#1746,#1745,#1584,.T.);
#2138=EDGE_CURVE('',#1746,#1747,#1123,.T.);
#2139=EDGE_CURVE('',#1748,#1747,#892,.T.);
#2140=EDGE_CURVE('',#1747,#1748,#893,.T.);
#2141=EDGE_CURVE('',#1749,#1745,#894,.T.);
#2142=EDGE_CURVE('',#1749,#1749,#1585,.T.);
#2143=EDGE_CURVE('',#1750,#1749,#290,.T.);
#2144=EDGE_CURVE('',#1750,#1750,#1586,.T.);
#2145=EDGE_CURVE('',#1748,#1751,#895,.T.);
#2146=EDGE_CURVE('',#1751,#1751,#896,.T.);
#2147=EDGE_CURVE('',#1752,#1752,#1587,.T.);
#2148=EDGE_CURVE('',#1752,#1753,#897,.T.);
#2149=EDGE_CURVE('',#1753,#1753,#1588,.T.);
#2150=EDGE_CURVE('',#1753,#1754,#291,.T.);
#2151=EDGE_CURVE('',#1754,#1754,#1589,.T.);
#2152=EDGE_CURVE('',#1754,#1755,#898,.T.);
#2153=EDGE_CURVE('',#1755,#1755,#1590,.T.);
#2154=EDGE_CURVE('',#1756,#1757,#899,.T.);
#2155=EDGE_CURVE('',#1757,#1756,#900,.T.);
#2156=EDGE_CURVE('',#1758,#1750,#901,.T.);
#2157=EDGE_CURVE('',#1758,#1758,#1591,.T.);
#2158=EDGE_CURVE('',#1759,#1759,#902,.T.);
#2159=EDGE_CURVE('',#1760,#1761,#903,.F.);
#2160=EDGE_CURVE('',#1761,#1762,#1124,.T.);
#2161=EDGE_CURVE('',#1762,#1763,#904,.T.);
#2162=EDGE_CURVE('',#1763,#1764,#1125,.T.);
#2163=EDGE_CURVE('',#1764,#1760,#1592,.F.);
#2164=EDGE_CURVE('',#1765,#1766,#905,.T.);
#2165=EDGE_CURVE('',#1766,#1763,#1593,.T.);
#2166=EDGE_CURVE('',#1762,#1765,#1594,.T.);
#2167=EDGE_CURVE('',#1767,#1768,#906,.T.);
#2168=EDGE_CURVE('',#1768,#1766,#1126,.T.);
#2169=EDGE_CURVE('',#1765,#1767,#1127,.T.);
#2170=EDGE_CURVE('',#1769,#1770,#907,.T.);
#2171=EDGE_CURVE('',#1770,#1768,#1595,.T.);
#2172=EDGE_CURVE('',#1767,#1769,#1596,.T.);
#2173=EDGE_CURVE('',#1756,#1771,#1597,.T.);
#2174=EDGE_CURVE('',#1756,#1770,#1128,.T.);
#2175=EDGE_CURVE('',#1769,#1771,#1129,.T.);
#2176=EDGE_CURVE('',#1772,#1761,#1130,.T.);
#2177=EDGE_CURVE('',#1771,#1772,#1598,.F.);
#2178=EDGE_CURVE('',#1757,#1773,#1599,.F.);
#2179=EDGE_CURVE('',#1773,#1774,#1131,.T.);
#2180=EDGE_CURVE('',#1774,#1775,#908,.T.);
#2181=EDGE_CURVE('',#1775,#1757,#1132,.T.);
#2182=EDGE_CURVE('',#1776,#1777,#909,.T.);
#2183=EDGE_CURVE('',#1777,#1775,#1600,.T.);
#2184=EDGE_CURVE('',#1774,#1776,#1601,.T.);
#2185=EDGE_CURVE('',#1778,#1779,#910,.T.);
#2186=EDGE_CURVE('',#1779,#1777,#1133,.T.);
#2187=EDGE_CURVE('',#1776,#1778,#1134,.T.);
#2188=EDGE_CURVE('',#1780,#1781,#911,.T.);
#2189=EDGE_CURVE('',#1781,#1779,#1602,.T.);
#2190=EDGE_CURVE('',#1778,#1780,#1603,.T.);
#2191=EDGE_CURVE('',#1782,#1783,#1604,.T.);
#2192=EDGE_CURVE('',#1782,#1781,#1135,.T.);
#2193=EDGE_CURVE('',#1780,#1784,#1136,.T.);
#2194=EDGE_CURVE('',#1783,#1784,#912,.T.);
#2195=EDGE_CURVE('',#1785,#1773,#1605,.F.);
#2196=EDGE_CURVE('',#1784,#1785,#1137,.T.);
#2197=EDGE_CURVE('',#1783,#1760,#913,.F.);
#2198=EDGE_CURVE('',#1764,#1782,#914,.T.);
#2199=EDGE_CURVE('',#1772,#1785,#915,.T.);
#2200=EDGE_CURVE('',#1770,#1775,#916,.T.);
#2201=EDGE_CURVE('',#1777,#1768,#917,.T.);
#2202=EDGE_CURVE('',#1766,#1779,#918,.T.);
#2203=EDGE_CURVE('',#1786,#1763,#919,.T.);
#2204=EDGE_CURVE('',#1786,#1787,#1138,.T.);
#2205=EDGE_CURVE('',#1788,#1787,#920,.T.);
#2206=EDGE_CURVE('',#1787,#1788,#921,.T.);
#2207=EDGE_CURVE('',#1781,#1786,#922,.T.);
#2208=EDGE_CURVE('',#1788,#1759,#923,.T.);
#2767=ORIENTED_EDGE('',*,*,#2136,.F.);
#2768=ORIENTED_EDGE('',*,*,#2137,.F.);
#2769=ORIENTED_EDGE('',*,*,#2138,.T.);
#2770=ORIENTED_EDGE('',*,*,#2139,.F.);
#2771=ORIENTED_EDGE('',*,*,#2140,.F.);
#2772=ORIENTED_EDGE('',*,*,#2138,.F.);
#2773=ORIENTED_EDGE('',*,*,#2136,.T.);
#2774=ORIENTED_EDGE('',*,*,#2137,.T.);
#2775=ORIENTED_EDGE('',*,*,#2141,.F.);
#2776=ORIENTED_EDGE('',*,*,#2142,.T.);
#2777=ORIENTED_EDGE('',*,*,#2141,.T.);
#2778=ORIENTED_EDGE('',*,*,#2142,.F.);
#2779=ORIENTED_EDGE('',*,*,#2143,.F.);
#2780=ORIENTED_EDGE('',*,*,#2144,.F.);
#2781=ORIENTED_EDGE('',*,*,#2143,.T.);
#2782=ORIENTED_EDGE('',*,*,#2140,.T.);
#2783=ORIENTED_EDGE('',*,*,#2145,.T.);
#2784=ORIENTED_EDGE('',*,*,#2146,.T.);
#2785=ORIENTED_EDGE('',*,*,#2145,.F.);
#2786=ORIENTED_EDGE('',*,*,#2139,.T.);
#2787=ORIENTED_EDGE('',*,*,#2147,.F.);
#2788=ORIENTED_EDGE('',*,*,#2146,.F.);
#2789=ORIENTED_EDGE('',*,*,#2148,.T.);
#2790=ORIENTED_EDGE('',*,*,#2149,.T.);
#2791=ORIENTED_EDGE('',*,*,#2148,.F.);
#2792=ORIENTED_EDGE('',*,*,#2147,.T.);
#2793=ORIENTED_EDGE('',*,*,#2149,.F.);
#2794=ORIENTED_EDGE('',*,*,#2150,.T.);
#2795=ORIENTED_EDGE('',*,*,#2151,.F.);
#2796=ORIENTED_EDGE('',*,*,#2150,.F.);
#2797=ORIENTED_EDGE('',*,*,#2152,.T.);
#2798=ORIENTED_EDGE('',*,*,#2153,.T.);
#2799=ORIENTED_EDGE('',*,*,#2152,.F.);
#2800=ORIENTED_EDGE('',*,*,#2151,.T.);
#2801=ORIENTED_EDGE('',*,*,#2154,.T.);
#2802=ORIENTED_EDGE('',*,*,#2155,.T.);
#2803=ORIENTED_EDGE('',*,*,#2153,.F.);
#2804=ORIENTED_EDGE('',*,*,#2156,.T.);
#2805=ORIENTED_EDGE('',*,*,#2144,.T.);
#2806=ORIENTED_EDGE('',*,*,#2156,.F.);
#2807=ORIENTED_EDGE('',*,*,#2157,.T.);
#2808=ORIENTED_EDGE('',*,*,#2158,.F.);
#2809=ORIENTED_EDGE('',*,*,#2157,.F.);
#2810=ORIENTED_EDGE('',*,*,#2159,.T.);
#2811=ORIENTED_EDGE('',*,*,#2160,.T.);
#2812=ORIENTED_EDGE('',*,*,#2161,.T.);
#2813=ORIENTED_EDGE('',*,*,#2162,.T.);
#2814=ORIENTED_EDGE('',*,*,#2163,.T.);
#2815=ORIENTED_EDGE('',*,*,#2164,.T.);
#2816=ORIENTED_EDGE('',*,*,#2165,.T.);
#2817=ORIENTED_EDGE('',*,*,#2161,.F.);
#2818=ORIENTED_EDGE('',*,*,#2166,.T.);
#2819=ORIENTED_EDGE('',*,*,#2167,.T.);
#2820=ORIENTED_EDGE('',*,*,#2168,.T.);
#2821=ORIENTED_EDGE('',*,*,#2164,.F.);
#2822=ORIENTED_EDGE('',*,*,#2169,.T.);
#2823=ORIENTED_EDGE('',*,*,#2170,.T.);
#2824=ORIENTED_EDGE('',*,*,#2171,.T.);
#2825=ORIENTED_EDGE('',*,*,#2167,.F.);
#2826=ORIENTED_EDGE('',*,*,#2172,.T.);
#2827=ORIENTED_EDGE('',*,*,#2173,.F.);
#2828=ORIENTED_EDGE('',*,*,#2174,.T.);
#2829=ORIENTED_EDGE('',*,*,#2170,.F.);
#2830=ORIENTED_EDGE('',*,*,#2175,.T.);
#2831=ORIENTED_EDGE('',*,*,#2175,.F.);
#2832=ORIENTED_EDGE('',*,*,#2172,.F.);
#2833=ORIENTED_EDGE('',*,*,#2169,.F.);
#2834=ORIENTED_EDGE('',*,*,#2166,.F.);
#2835=ORIENTED_EDGE('',*,*,#2160,.F.);
#2836=ORIENTED_EDGE('',*,*,#2176,.F.);
#2837=ORIENTED_EDGE('',*,*,#2177,.F.);
#2838=ORIENTED_EDGE('',*,*,#2178,.T.);
#2839=ORIENTED_EDGE('',*,*,#2179,.T.);
#2840=ORIENTED_EDGE('',*,*,#2180,.T.);
#2841=ORIENTED_EDGE('',*,*,#2181,.T.);
#2842=ORIENTED_EDGE('',*,*,#2182,.T.);
#2843=ORIENTED_EDGE('',*,*,#2183,.T.);
#2844=ORIENTED_EDGE('',*,*,#2180,.F.);
#2845=ORIENTED_EDGE('',*,*,#2184,.T.);
#2846=ORIENTED_EDGE('',*,*,#2185,.T.);
#2847=ORIENTED_EDGE('',*,*,#2186,.T.);
#2848=ORIENTED_EDGE('',*,*,#2182,.F.);
#2849=ORIENTED_EDGE('',*,*,#2187,.T.);
#2850=ORIENTED_EDGE('',*,*,#2188,.T.);
#2851=ORIENTED_EDGE('',*,*,#2189,.T.);
#2852=ORIENTED_EDGE('',*,*,#2185,.F.);
#2853=ORIENTED_EDGE('',*,*,#2190,.T.);
#2854=ORIENTED_EDGE('',*,*,#2191,.F.);
#2855=ORIENTED_EDGE('',*,*,#2192,.T.);
#2856=ORIENTED_EDGE('',*,*,#2188,.F.);
#2857=ORIENTED_EDGE('',*,*,#2193,.T.);
#2858=ORIENTED_EDGE('',*,*,#2194,.F.);
#2859=ORIENTED_EDGE('',*,*,#2193,.F.);
#2860=ORIENTED_EDGE('',*,*,#2190,.F.);
#2861=ORIENTED_EDGE('',*,*,#2187,.F.);
#2862=ORIENTED_EDGE('',*,*,#2184,.F.);
#2863=ORIENTED_EDGE('',*,*,#2179,.F.);
#2864=ORIENTED_EDGE('',*,*,#2195,.F.);
#2865=ORIENTED_EDGE('',*,*,#2196,.F.);
#2866=ORIENTED_EDGE('',*,*,#2197,.T.);
#2867=ORIENTED_EDGE('',*,*,#2163,.F.);
#2868=ORIENTED_EDGE('',*,*,#2198,.T.);
#2869=ORIENTED_EDGE('',*,*,#2191,.T.);
#2870=ORIENTED_EDGE('',*,*,#2197,.F.);
#2871=ORIENTED_EDGE('',*,*,#2194,.T.);
#2872=ORIENTED_EDGE('',*,*,#2196,.T.);
#2873=ORIENTED_EDGE('',*,*,#2199,.F.);
#2874=ORIENTED_EDGE('',*,*,#2176,.T.);
#2875=ORIENTED_EDGE('',*,*,#2159,.F.);
#2876=ORIENTED_EDGE('',*,*,#2177,.T.);
#2877=ORIENTED_EDGE('',*,*,#2199,.T.);
#2878=ORIENTED_EDGE('',*,*,#2195,.T.);
#2879=ORIENTED_EDGE('',*,*,#2178,.F.);
#2880=ORIENTED_EDGE('',*,*,#2154,.F.);
#2881=ORIENTED_EDGE('',*,*,#2173,.T.);
#2882=ORIENTED_EDGE('',*,*,#2174,.F.);
#2883=ORIENTED_EDGE('',*,*,#2155,.F.);
#2884=ORIENTED_EDGE('',*,*,#2181,.F.);
#2885=ORIENTED_EDGE('',*,*,#2200,.F.);
#2886=ORIENTED_EDGE('',*,*,#2171,.F.);
#2887=ORIENTED_EDGE('',*,*,#2200,.T.);
#2888=ORIENTED_EDGE('',*,*,#2183,.F.);
#2889=ORIENTED_EDGE('',*,*,#2201,.T.);
#2890=ORIENTED_EDGE('',*,*,#2168,.F.);
#2891=ORIENTED_EDGE('',*,*,#2201,.F.);
#2892=ORIENTED_EDGE('',*,*,#2186,.F.);
#2893=ORIENTED_EDGE('',*,*,#2202,.F.);
#2894=ORIENTED_EDGE('',*,*,#2162,.F.);
#2895=ORIENTED_EDGE('',*,*,#2203,.F.);
#2896=ORIENTED_EDGE('',*,*,#2204,.T.);
#2897=ORIENTED_EDGE('',*,*,#2205,.F.);
#2898=ORIENTED_EDGE('',*,*,#2206,.F.);
#2899=ORIENTED_EDGE('',*,*,#2204,.F.);
#2900=ORIENTED_EDGE('',*,*,#2207,.F.);
#2901=ORIENTED_EDGE('',*,*,#2192,.F.);
#2902=ORIENTED_EDGE('',*,*,#2198,.F.);
#2903=ORIENTED_EDGE('',*,*,#2165,.F.);
#2904=ORIENTED_EDGE('',*,*,#2202,.T.);
#2905=ORIENTED_EDGE('',*,*,#2189,.F.);
#2906=ORIENTED_EDGE('',*,*,#2207,.T.);
#2907=ORIENTED_EDGE('',*,*,#2203,.T.);
#2908=ORIENTED_EDGE('',*,*,#2205,.T.);
#2909=ORIENTED_EDGE('',*,*,#2206,.T.);
#2910=ORIENTED_EDGE('',*,*,#2208,.T.);
#2911=ORIENTED_EDGE('',*,*,#2158,.T.);
#2912=ORIENTED_EDGE('',*,*,#2208,.F.);
#4029=CYLINDRICAL_SURFACE('',#4507,11.05);
#4030=CYLINDRICAL_SURFACE('',#4523,0.5);
#4031=CYLINDRICAL_SURFACE('',#4527,0.5);
#4032=CYLINDRICAL_SURFACE('',#4530,0.5);
#4033=CYLINDRICAL_SURFACE('',#4532,0.5);
#4034=CYLINDRICAL_SURFACE('',#4535,0.5);
#4035=CYLINDRICAL_SURFACE('',#4538,0.5);
#4036=CYLINDRICAL_SURFACE('',#4547,57.5);
#4037=CYLINDRICAL_SURFACE('',#4553,60.5);
#4114=ADVANCED_FACE('',(#324),#4029,.F.);
#4115=ADVANCED_FACE('',(#325),#298,.F.);
#4116=ADVANCED_FACE('',(#326),#294,.T.);
#4117=ADVANCED_FACE('',(#327),#258,.T.);
#4118=ADVANCED_FACE('',(#328,#141),#169,.T.);
#4119=ADVANCED_FACE('',(#329),#299,.F.);
#4120=ADVANCED_FACE('',(#330),#295,.T.);
#4121=ADVANCED_FACE('',(#331),#300,.T.);
#4122=ADVANCED_FACE('',(#332,#142),#170,.T.);
#4123=ADVANCED_FACE('',(#333),#301,.F.);
#4124=ADVANCED_FACE('',(#334,#143),#171,.T.);
#4125=ADVANCED_FACE('',(#335),#4030,.T.);
#4126=ADVANCED_FACE('',(#336),#302,.F.);
#4127=ADVANCED_FACE('',(#337),#4031,.T.);
#4128=ADVANCED_FACE('',(#338),#303,.F.);
#4129=ADVANCED_FACE('',(#339),#4032,.T.);
#4130=ADVANCED_FACE('',(#340),#172,.F.);
#4131=ADVANCED_FACE('',(#341),#4033,.T.);
#4132=ADVANCED_FACE('',(#342),#304,.F.);
#4133=ADVANCED_FACE('',(#343),#4034,.T.);
#4134=ADVANCED_FACE('',(#344),#305,.F.);
#4135=ADVANCED_FACE('',(#345),#4035,.T.);
#4136=ADVANCED_FACE('',(#346),#173,.F.);
#4137=ADVANCED_FACE('',(#347),#259,.T.);
#4138=ADVANCED_FACE('',(#348),#174,.F.);
#4139=ADVANCED_FACE('',(#349),#260,.T.);
#4140=ADVANCED_FACE('',(#350),#4036,.F.);
#4141=ADVANCED_FACE('',(#351),#261,.T.);
#4142=ADVANCED_FACE('',(#352),#175,.T.);
#4143=ADVANCED_FACE('',(#353),#4037,.T.);
#4144=ADVANCED_FACE('',(#354),#262,.T.);
#4145=ADVANCED_FACE('',(#355),#263,.T.);
#4384=CLOSED_SHELL('',(#4114,#4115,#4116,#4117,#4118,#4119,#4120,#4121,
#4122,#4123,#4124,#4125,#4126,#4127,#4128,#4129,#4130,#4131,#4132,#4133,
#4134,#4135,#4136,#4137,#4138,#4139,#4140,#4141,#4142,#4143,#4144,#4145));
#4506=AXIS2_PLACEMENT_3D('',#6233,#5006,#5007);
#4507=AXIS2_PLACEMENT_3D('',#6234,#5008,#5009);
#4508=AXIS2_PLACEMENT_3D('',#6287,#5011,#5012);
#4509=AXIS2_PLACEMENT_3D('',#6288,#5013,#5014);
#4510=AXIS2_PLACEMENT_3D('',#6358,#5015,#5016);
#4511=AXIS2_PLACEMENT_3D('',#6696,#5017,#5018);
#4512=AXIS2_PLACEMENT_3D('',#6698,#5019,#5020);
#4513=AXIS2_PLACEMENT_3D('',#6699,#5021,#5022);
#4514=AXIS2_PLACEMENT_3D('',#6700,#5023,#5024);
#4515=AXIS2_PLACEMENT_3D('',#6788,#5025,#5026);
#4516=AXIS2_PLACEMENT_3D('',#7203,#5027,#5028);
#4517=AXIS2_PLACEMENT_3D('',#7223,#5029,#5030);
#4518=AXIS2_PLACEMENT_3D('',#7226,#5031,#5032);
#4519=AXIS2_PLACEMENT_3D('',#7227,#5033,#5034);
#4520=AXIS2_PLACEMENT_3D('',#7305,#5035,#5036);
#4521=AXIS2_PLACEMENT_3D('',#7355,#5037,#5038);
#4522=AXIS2_PLACEMENT_3D('',#7357,#5039,#5040);
#4523=AXIS2_PLACEMENT_3D('',#7358,#5041,#5042);
#4524=AXIS2_PLACEMENT_3D('',#7361,#5043,#5044);
#4525=AXIS2_PLACEMENT_3D('',#7365,#5046,#5047);
#4526=AXIS2_PLACEMENT_3D('',#7409,#5049,#5050);
#4527=AXIS2_PLACEMENT_3D('',#7420,#5051,#5052);
#4528=AXIS2_PLACEMENT_3D('',#7423,#5053,#5054);
#4529=AXIS2_PLACEMENT_3D('',#7453,#5057,#5058);
#4530=AXIS2_PLACEMENT_3D('',#7464,#5059,#5060);
#4531=AXIS2_PLACEMENT_3D('',#7482,#5063,#5064);
#4532=AXIS2_PLACEMENT_3D('',#7489,#5066,#5067);
#4533=AXIS2_PLACEMENT_3D('',#7508,#5069,#5070);
#4534=AXIS2_PLACEMENT_3D('',#7537,#5072,#5073);
#4535=AXIS2_PLACEMENT_3D('',#7548,#5074,#5075);
#4536=AXIS2_PLACEMENT_3D('',#7551,#5076,#5077);
#4537=AXIS2_PLACEMENT_3D('',#7581,#5080,#5081);
#4538=AXIS2_PLACEMENT_3D('',#7592,#5082,#5083);
#4539=AXIS2_PLACEMENT_3D('',#7612,#5086,#5087);
#4540=AXIS2_PLACEMENT_3D('',#7613,#5088,#5089);
#4541=AXIS2_PLACEMENT_3D('',#7620,#5091,#5092);
#4542=AXIS2_PLACEMENT_3D('',#7621,#5093,#5094);
#4543=AXIS2_PLACEMENT_3D('',#7622,#5095,#5096);
#4544=AXIS2_PLACEMENT_3D('',#7623,#5097,#5098);
#4545=AXIS2_PLACEMENT_3D('',#7624,#5099,#5100);
#4546=AXIS2_PLACEMENT_3D('',#7625,#5101,#5102);
#4547=AXIS2_PLACEMENT_3D('',#7626,#5103,#5104);
#4548=AXIS2_PLACEMENT_3D('',#7627,#5105,#5106);
#4549=AXIS2_PLACEMENT_3D('',#7628,#5107,#5108);
#4550=AXIS2_PLACEMENT_3D('',#7629,#5109,#5110);
#4551=AXIS2_PLACEMENT_3D('',#7630,#5111,#5112);
#4552=AXIS2_PLACEMENT_3D('',#7631,#5113,#5114);
#4553=AXIS2_PLACEMENT_3D('',#7632,#5115,#5116);
#4554=AXIS2_PLACEMENT_3D('',#7634,#5117,#5118);
#4555=AXIS2_PLACEMENT_3D('',#7638,#5120,#5121);
#4556=AXIS2_PLACEMENT_3D('',#7639,#5122,#5123);
#4557=AXIS2_PLACEMENT_3D('',#7640,#5124,#5125);
#4558=AXIS2_PLACEMENT_3D('',#7641,#5126,#5127);
#4559=AXIS2_PLACEMENT_3D('',#7642,#5128,#5129);
#4560=AXIS2_PLACEMENT_3D('',#7643,#5130,#5131);
#5006=DIRECTION('axis',(0.,0.,1.));
#5007=DIRECTION('refdir',(1.,0.,0.));
#5008=DIRECTION('center_axis',(1.,0.,0.));
#5009=DIRECTION('ref_axis',(0.,1.,0.));
#5010=DIRECTION('',(1.,0.,0.));
#5011=DIRECTION('center_axis',(-1.,0.,0.));
#5012=DIRECTION('ref_axis',(0.,1.,0.));
#5013=DIRECTION('center_axis',(-1.,0.,0.));
#5014=DIRECTION('ref_axis',(0.,1.,0.));
#5015=DIRECTION('center_axis',(1.48334715740448E-15,-5.5511151231258E-16,
1.));
#5016=DIRECTION('ref_axis',(-0.989545127054242,-0.144223581716739,1.38777878078145E-15));
#5017=DIRECTION('center_axis',(1.,0.,0.));
#5018=DIRECTION('ref_axis',(0.,0.,-1.));
#5019=DIRECTION('center_axis',(0.,-1.,-1.22464679914735E-16));
#5020=DIRECTION('ref_axis',(0.,-1.22464679914735E-16,1.));
#5021=DIRECTION('center_axis',(1.,0.,0.));
#5022=DIRECTION('ref_axis',(0.,-1.,1.83697019872103E-16));
#5023=DIRECTION('center_axis',(1.,0.,0.));
#5024=DIRECTION('ref_axis',(0.,0.,-1.));
#5025=DIRECTION('center_axis',(0.,1.03326339950577E-13,1.));
#5026=DIRECTION('ref_axis',(1.,0.,0.));
#5027=DIRECTION('center_axis',(0.,-3.49549273361196E-12,-1.));
#5028=DIRECTION('ref_axis',(-0.999873892461117,-0.0158807800392414,5.5511151231258E-14));
#5029=DIRECTION('center_axis',(1.,0.,0.));
#5030=DIRECTION('ref_axis',(0.,0.,-1.));
#5031=DIRECTION('center_axis',(1.,0.,0.));
#5032=DIRECTION('ref_axis',(0.,0.,-1.));
#5033=DIRECTION('center_axis',(1.,0.,0.));
#5034=DIRECTION('ref_axis',(0.,0.,-1.));
#5035=DIRECTION('center_axis',(0.,6.17228125957411E-12,1.));
#5036=DIRECTION('ref_axis',(-1.,0.,0.));
#5037=DIRECTION('center_axis',(-1.,0.,0.));
#5038=DIRECTION('ref_axis',(0.,0.,1.));
#5039=DIRECTION('center_axis',(1.,0.,0.));
#5040=DIRECTION('ref_axis',(0.,-1.,1.83697019872103E-16));
#5041=DIRECTION('center_axis',(1.,0.,0.));
#5042=DIRECTION('ref_axis',(0.,0.724568837309466,0.689202437604517));
#5043=DIRECTION('center_axis',(-1.,0.,0.));
#5044=DIRECTION('ref_axis',(0.,0.724568837309466,0.689202437604517));
#5045=DIRECTION('',(1.,0.,0.));
#5046=DIRECTION('center_axis',(-1.,0.,0.));
#5047=DIRECTION('ref_axis',(0.,0.,1.));
#5048=DIRECTION('',(-1.,0.,0.));
#5049=DIRECTION('center_axis',(0.,1.,0.));
#5050=DIRECTION('ref_axis',(0.,0.,1.));
#5051=DIRECTION('center_axis',(0.,-1.,0.));
#5052=DIRECTION('ref_axis',(0.707106781186553,0.,0.707106781186542));
#5053=DIRECTION('center_axis',(0.,1.,0.));
#5054=DIRECTION('ref_axis',(0.,0.,1.));
#5055=DIRECTION('',(0.,1.,0.));
#5056=DIRECTION('',(0.,-1.,0.));
#5057=DIRECTION('center_axis',(1.,0.,0.));
#5058=DIRECTION('ref_axis',(0.,0.,1.));
#5059=DIRECTION('center_axis',(-1.,0.,0.));
#5060=DIRECTION('ref_axis',(0.,-0.688576743024685,0.725163477407348));
#5061=DIRECTION('',(1.,0.,0.));
#5062=DIRECTION('',(-1.,0.,0.));
#5063=DIRECTION('center_axis',(0.,0.,-1.));
#5064=DIRECTION('ref_axis',(-1.,0.,0.));
#5065=DIRECTION('',(0.,1.,0.));
#5066=DIRECTION('center_axis',(1.,0.,0.));
#5067=DIRECTION('ref_axis',(0.,-0.688576743024685,-0.725163477407348));
#5068=DIRECTION('',(1.,0.,0.));
#5069=DIRECTION('center_axis',(-1.,0.,0.));
#5070=DIRECTION('ref_axis',(0.,0.,-1.));
#5071=DIRECTION('',(-1.,0.,0.));
#5072=DIRECTION('center_axis',(0.,-1.,0.));
#5073=DIRECTION('ref_axis',(0.,0.,-1.));
#5074=DIRECTION('center_axis',(0.,1.,0.));
#5075=DIRECTION('ref_axis',(0.707106781186553,0.,-0.707106781186542));
#5076=DIRECTION('center_axis',(0.,-1.,0.));
#5077=DIRECTION('ref_axis',(0.,0.,-1.));
#5078=DIRECTION('',(0.,-1.,0.));
#5079=DIRECTION('',(0.,1.,0.));
#5080=DIRECTION('center_axis',(1.,0.,0.));
#5081=DIRECTION('ref_axis',(0.,0.,-1.));
#5082=DIRECTION('center_axis',(-1.,0.,0.));
#5083=DIRECTION('ref_axis',(0.,0.724568837309466,-0.689202437604517));
#5084=DIRECTION('',(1.,0.,0.));
#5085=DIRECTION('',(-1.,0.,0.));
#5086=DIRECTION('center_axis',(-1.,0.,0.));
#5087=DIRECTION('ref_axis',(0.,0.724568837309466,-0.689202437604517));
#5088=DIRECTION('center_axis',(0.,0.,1.));
#5089=DIRECTION('ref_axis',(1.,0.,0.));
#5090=DIRECTION('',(0.,-1.,0.));
#5091=DIRECTION('center_axis',(-1.,0.,0.));
#5092=DIRECTION('ref_axis',(0.,0.,1.));
#5093=DIRECTION('center_axis',(1.,0.,0.));
#5094=DIRECTION('ref_axis',(0.,0.,1.));
#5095=DIRECTION('center_axis',(1.,0.,0.));
#5096=DIRECTION('ref_axis',(0.,1.,0.));
#5097=DIRECTION('center_axis',(-1.,0.,0.));
#5098=DIRECTION('ref_axis',(0.,-1.,0.));
#5099=DIRECTION('center_axis',(1.,0.,0.));
#5100=DIRECTION('ref_axis',(0.,1.,0.));
#5101=DIRECTION('center_axis',(1.,0.,0.));
#5102=DIRECTION('ref_axis',(0.,0.,-1.));
#5103=DIRECTION('center_axis',(1.,0.,0.));
#5104=DIRECTION('ref_axis',(0.,-1.,-1.22464679914735E-16));
#5105=DIRECTION('center_axis',(-1.,0.,0.));
#5106=DIRECTION('ref_axis',(0.,-1.,1.83697019872103E-16));
#5107=DIRECTION('center_axis',(1.,0.,0.));
#5108=DIRECTION('ref_axis',(0.,-1.,-6.12323399573677E-17));
#5109=DIRECTION('center_axis',(1.,0.,0.));
#5110=DIRECTION('ref_axis',(0.,-1.,1.83697019872103E-16));
#5111=DIRECTION('center_axis',(1.,0.,0.));
#5112=DIRECTION('ref_axis',(0.,0.,-1.));
#5113=DIRECTION('center_axis',(-1.,0.,0.));
#5114=DIRECTION('ref_axis',(0.,-1.,1.83697019872103E-16));
#5115=DIRECTION('center_axis',(1.,0.,0.));
#5116=DIRECTION('ref_axis',(0.,1.,0.));
#5117=DIRECTION('center_axis',(1.,0.,0.));
#5118=DIRECTION('ref_axis',(0.,-1.,1.83697019872103E-16));
#5119=DIRECTION('',(-1.,0.,0.));
#5120=DIRECTION('center_axis',(-1.,0.,0.));
#5121=DIRECTION('ref_axis',(0.,-1.,1.83697019872103E-16));
#5122=DIRECTION('center_axis',(-1.,0.,0.));
#5123=DIRECTION('ref_axis',(0.,-1.,1.83697019872103E-16));
#5124=DIRECTION('center_axis',(1.,0.,0.));
#5125=DIRECTION('ref_axis',(0.,-1.,1.83697019872103E-16));
#5126=DIRECTION('center_axis',(1.,0.,0.));
#5127=DIRECTION('ref_axis',(0.,-1.,-6.12323399573677E-17));
#5128=DIRECTION('center_axis',(1.,0.,0.));
#5129=DIRECTION('ref_axis',(0.,0.,-1.));
#5130=DIRECTION('center_axis',(0.,-1.,-1.22464679914735E-16));
#5131=DIRECTION('ref_axis',(0.,-1.22464679914735E-16,1.));
#6233=CARTESIAN_POINT('',(0.,0.,0.));
#6234=CARTESIAN_POINT('Origin',(65.75,0.,0.));
#6235=CARTESIAN_POINT('',(65.2272111655667,11.05,-4.81623674987417E-16));
#6236=CARTESIAN_POINT('',(65.2272111655668,-11.0491603167577,0.000511766293852513));
#6237=CARTESIAN_POINT('Ctrl Pts',(65.2272111655667,11.05,-8.04843840616275E-16));
#6238=CARTESIAN_POINT('Ctrl Pts',(65.2272111655667,11.05,1.65300226112955));
#6239=CARTESIAN_POINT('Ctrl Pts',(65.2272111655667,10.6732111658624,3.30528105206125));
#6240=CARTESIAN_POINT('Ctrl Pts',(65.2272111655667,9.95613525638491,4.79448116918521));
#6241=CARTESIAN_POINT('Ctrl Pts',(65.2272111655667,9.2390593469074,6.28368128630917));
#6242=CARTESIAN_POINT('Ctrl Pts',(65.2272111655667,8.18169636208996,7.60980272962538));
#6243=CARTESIAN_POINT('Ctrl Pts',(65.2272111655667,6.88961460043875,8.63998814917286));
#6244=CARTESIAN_POINT('Ctrl Pts',(65.2272111655667,5.59753283878755,9.67017356872034));
#6245=CARTESIAN_POINT('Ctrl Pts',(65.2272111655667,4.07073230030258,10.4044229644991));
#6246=CARTESIAN_POINT('Ctrl Pts',(65.2272111655667,2.45913707576071,10.7727896191196));
#6247=CARTESIAN_POINT('Ctrl Pts',(65.2272111655667,0.847541851218851,11.14115627374));
#6248=CARTESIAN_POINT('Ctrl Pts',(65.2272111655667,-0.848848059379907,11.1436401872022));
#6249=CARTESIAN_POINT('Ctrl Pts',(65.2272111655667,-2.45957472900739,10.7749338027229));
#6250=CARTESIAN_POINT('Ctrl Pts',(65.2272111655667,-4.6072102885107,10.2833252900838));
#6251=CARTESIAN_POINT('Ctrl Pts',(65.2272111655668,-6.60255564184286,9.13182291443765));
#6252=CARTESIAN_POINT('Ctrl Pts',(65.2272111655667,-8.10144894371101,7.51774250750075));
#6253=CARTESIAN_POINT('Ctrl Pts',(65.2272111655667,-8.85089559464509,6.7107023040323));
#6254=CARTESIAN_POINT('Ctrl Pts',(65.2272111655667,-9.47622923271317,5.78801759274117));
#6255=CARTESIAN_POINT('Ctrl Pts',(65.2272111655667,-9.95481493068238,4.79417459098899));
#6256=CARTESIAN_POINT('Ctrl Pts',(65.2272111655667,-10.4334006286516,3.80033158923682));
#6257=CARTESIAN_POINT('Ctrl Pts',(65.2272111655667,-10.7652383865219,2.7353302970236));
#6258=CARTESIAN_POINT('Ctrl Pts',(65.2272111655667,-10.9288653221363,1.64620606893596));
#6259=CARTESIAN_POINT('Ctrl Pts',(65.2272111655667,-11.0106742828143,1.10167395498666));
#6260=CARTESIAN_POINT('Ctrl Pts',(65.2272111655667,-11.0504351711937,0.551111771520428));
#6261=CARTESIAN_POINT('Ctrl Pts',(65.2272111655667,-11.0491603167577,0.000511766293852513));
#6262=CARTESIAN_POINT('Ctrl Pts',(65.2272111655668,-11.0491603167577,0.000511766293852513));
#6263=CARTESIAN_POINT('Ctrl Pts',(65.2272111655667,-11.0453354725056,-1.6514095869656));
#6264=CARTESIAN_POINT('Ctrl Pts',(65.2272111655667,-10.6721346818115,-3.30367138607943));
#6265=CARTESIAN_POINT('Ctrl Pts',(65.2272111655667,-9.95689686460624,-4.79444728464091));
#6266=CARTESIAN_POINT('Ctrl Pts',(65.2272111655667,-9.48008040912453,-5.78827963350521));
#6267=CARTESIAN_POINT('Ctrl Pts',(65.2272111655667,-8.85125308035079,-6.71034310688341));
#6268=CARTESIAN_POINT('Ctrl Pts',(65.2272111655667,-8.1003801793731,-7.51685624327848));
#6269=CARTESIAN_POINT('Ctrl Pts',(65.2272111655667,-6.59863437741774,-9.12988251606863));
#6270=CARTESIAN_POINT('Ctrl Pts',(65.2272111655667,-4.60870628664658,-10.2807074409263));
#6271=CARTESIAN_POINT('Ctrl Pts',(65.2272111655667,-2.46069090561872,-10.7753211533687));
#6272=CARTESIAN_POINT('Ctrl Pts',(65.2272111655667,-1.38668321510479,-11.0226280095899));
#6273=CARTESIAN_POINT('Ctrl Pts',(65.2272111655667,-0.273153702026687,-11.1058820627073));
#6274=CARTESIAN_POINT('Ctrl Pts',(65.2272111655667,0.826207461938887,-11.0215937869587));
#6275=CARTESIAN_POINT('Ctrl Pts',(65.2272111655668,3.02492978987003,-10.8530172354614));
#6276=CARTESIAN_POINT('Ctrl Pts',(65.2272111655668,5.16697872135103,-10.0142713685));
#6277=CARTESIAN_POINT('Ctrl Pts',(65.2272111655668,6.89007612693015,-8.64177550465633));
#6278=CARTESIAN_POINT('Ctrl Pts',(65.2272111655668,8.1823991811145,-7.61240360677354));
#6279=CARTESIAN_POINT('Ctrl Pts',(65.2272111655667,9.23906200197904,-6.28279733564443));
#6280=CARTESIAN_POINT('Ctrl Pts',(65.2272111655667,9.95596220670041,-4.79294699923343));
#6281=CARTESIAN_POINT('Ctrl Pts',(65.2272111655667,10.6728624114218,-3.30309666282243));
#6282=CARTESIAN_POINT('Ctrl Pts',(65.2272111655667,11.05,-1.65300226112955));
#6283=CARTESIAN_POINT('Ctrl Pts',(65.2272111655667,11.05,-1.11022302462423E-15));
#6284=CARTESIAN_POINT('',(66.717944947177,-11.05,1.35323471305783E-15));
#6285=CARTESIAN_POINT('',(65.75,-11.05,-1.35323471305783E-15));
#6286=CARTESIAN_POINT('',(66.717944947177,-1.35323471305783E-15,11.05));
#6287=CARTESIAN_POINT('Origin',(66.717944947177,0.,0.));
#6288=CARTESIAN_POINT('Origin',(66.717944947177,0.,0.));
#6289=CARTESIAN_POINT('Ctrl Pts',(65.2272111655675,11.0499999999996,-8.04843840616481E-16));
#6290=CARTESIAN_POINT('Ctrl Pts',(65.2272111655675,11.0499999999996,1.65300226112949));
#6291=CARTESIAN_POINT('Ctrl Pts',(65.2272111655675,10.2964223317245,4.95755984299279));
#6292=CARTESIAN_POINT('Ctrl Pts',(65.2272111655675,7.12433337727229,8.9359241729413));
#6293=CARTESIAN_POINT('Ctrl Pts',(65.2272111655675,2.54393176181752,11.1386723602775));
#6294=CARTESIAN_POINT('Ctrl Pts',(65.2272111655675,-3.11070127351147,11.1469520718181));
#6295=CARTESIAN_POINT('Ctrl Pts',(65.2272111655675,-7.60022831850869,8.55607172661427));
#6296=CARTESIAN_POINT('Ctrl Pts',(65.2272111655675,-10.1015628707809,4.86533288144987));
#6297=CARTESIAN_POINT('Ctrl Pts',(65.2272111655675,-11.4289139022623,0.605327712597159));
#6298=CARTESIAN_POINT('Ctrl Pts',(65.2272111655675,-10.7377350666716,-3.94415268674868));
#6299=CARTESIAN_POINT('Ctrl Pts',(65.2272111655675,-7.59359842280306,-8.55447005363952));
#6300=CARTESIAN_POINT('Ctrl Pts',(65.2272111655675,-3.61374224126088,-10.8561199033547));
#6301=CARTESIAN_POINT('Ctrl Pts',(65.2272111655675,1.95390532412946,-11.2723901689417));
#6302=CARTESIAN_POINT('Ctrl Pts',(65.2272111655675,6.77351541996157,-9.3852119682787));
#6303=CARTESIAN_POINT('Ctrl Pts',(65.2272111655675,10.2957248228432,-4.95319106451515));
#6304=CARTESIAN_POINT('Ctrl Pts',(65.2272111655675,11.0499999999996,-1.65300226112949));
#6305=CARTESIAN_POINT('Ctrl Pts',(65.2272111655675,11.0499999999996,-1.40162863026563E-15));
#6306=CARTESIAN_POINT('Ctrl Pts',(65.0809549842406,11.1208351015851,-7.65476926691726E-16));
#6307=CARTESIAN_POINT('Ctrl Pts',(65.0809549842406,11.1208351015851,1.66346926418635));
#6308=CARTESIAN_POINT('Ctrl Pts',(65.0809549842406,10.3623404117656,4.98933947213189));
#6309=CARTESIAN_POINT('Ctrl Pts',(65.0809549842406,7.16993389260531,8.99309464113236));
#6310=CARTESIAN_POINT('Ctrl Pts',(65.0809549842406,2.5601655446675,11.2100133239775));
#6311=CARTESIAN_POINT('Ctrl Pts',(65.0809549842406,-3.1306002334161,11.2182832653346));
#6312=CARTESIAN_POINT('Ctrl Pts',(65.0809549842406,-7.64889972369121,8.61085072005576));
#6313=CARTESIAN_POINT('Ctrl Pts',(65.0809549842406,-10.1662171602437,4.89646684843357));
#6314=CARTESIAN_POINT('Ctrl Pts',(65.0809549842406,-11.5020966787491,0.609220450083247));
#6315=CARTESIAN_POINT('Ctrl Pts',(65.0809549842406,-10.8064244099587,-3.96945703932799));
#6316=CARTESIAN_POINT('Ctrl Pts',(65.0809549842406,-7.64230494153489,-8.60917577599024));
#6317=CARTESIAN_POINT('Ctrl Pts',(65.0809549842406,-3.63683147635714,-10.9256030117343));
#6318=CARTESIAN_POINT('Ctrl Pts',(65.0809549842406,1.96642553185435,-11.3445597508395));
#6319=CARTESIAN_POINT('Ctrl Pts',(65.0809549842406,6.81683558342508,-9.44530445284557));
#6320=CARTESIAN_POINT('Ctrl Pts',(65.0809549842406,10.361637717681,-4.98493807774593));
#6321=CARTESIAN_POINT('Ctrl Pts',(65.0809549842406,11.1208351015851,-1.66346926418635));
#6322=CARTESIAN_POINT('Ctrl Pts',(65.0809549842406,11.1208351015851,-1.22466367006471E-15));
#6323=CARTESIAN_POINT('Ctrl Pts',(64.9738208717935,11.26708032966,-6.84261163180322E-16));
#6324=CARTESIAN_POINT('Ctrl Pts',(64.9738208717935,11.26708032966,1.68537120997538));
#6325=CARTESIAN_POINT('Ctrl Pts',(64.9738208717935,10.4986285999894,5.05495216898997));
#6326=CARTESIAN_POINT('Ctrl Pts',(64.9738208717935,7.26423670697669,9.11138183115333));
#6327=CARTESIAN_POINT('Ctrl Pts',(64.9738208717935,2.59384822348416,11.3574440526352));
#6328=CARTESIAN_POINT('Ctrl Pts',(64.9738208717935,-3.17177793453904,11.3658355627214));
#6329=CARTESIAN_POINT('Ctrl Pts',(64.9738208717935,-7.74949708797367,8.72410231053509));
#6330=CARTESIAN_POINT('Ctrl Pts',(64.9738208717935,-10.299929206767,4.96086932020551));
#6331=CARTESIAN_POINT('Ctrl Pts',(64.9738208717935,-11.6533722919867,0.617229526149155));
#6332=CARTESIAN_POINT('Ctrl Pts',(64.9738208717935,-10.9485643243391,-4.0216534100572));
#6333=CARTESIAN_POINT('Ctrl Pts',(64.9738208717935,-7.74279975532283,-8.72241818640559));
#6334=CARTESIAN_POINT('Ctrl Pts',(64.9738208717935,-3.68467342228032,-11.0693030819176));
#6335=CARTESIAN_POINT('Ctrl Pts',(64.9738208717935,1.99228617997655,-11.4937656657012));
#6336=CARTESIAN_POINT('Ctrl Pts',(64.9738208717935,6.90650137190516,-9.56952991364493));
#6337=CARTESIAN_POINT('Ctrl Pts',(64.9738208717935,10.4979168106424,-5.05049383381464));
#6338=CARTESIAN_POINT('Ctrl Pts',(64.9738208717935,11.26708032966,-1.68537120997538));
#6339=CARTESIAN_POINT('Ctrl Pts',(64.9738208717935,11.26708032966,-8.59329092798487E-16));
#6340=CARTESIAN_POINT('Ctrl Pts',(64.9503835492166,11.4278882091416,-5.94987561328448E-16));
#6341=CARTESIAN_POINT('Ctrl Pts',(64.9503835492166,11.4278882091416,1.70953167870107));
#6342=CARTESIAN_POINT('Ctrl Pts',(64.9503835492166,10.6485396706842,5.12709861319939));
#6343=CARTESIAN_POINT('Ctrl Pts',(64.9503835492166,7.36797152942324,9.24151515780478));
#6344=CARTESIAN_POINT('Ctrl Pts',(64.9503835492167,2.63092921137885,11.519592989277));
#6345=CARTESIAN_POINT('Ctrl Pts',(64.9503835492166,-3.21708112269002,11.5281558506245));
#6346=CARTESIAN_POINT('Ctrl Pts',(64.9503835492167,-7.86014113917398,8.84867250689127));
#6347=CARTESIAN_POINT('Ctrl Pts',(64.9503835492167,-10.4470164004438,5.03171767144541));
#6348=CARTESIAN_POINT('Ctrl Pts',(64.9503835492166,-11.8197602196346,0.6260287266476));
#6349=CARTESIAN_POINT('Ctrl Pts',(64.9503835492166,-11.1049444308876,-4.0790349306743));
#6350=CARTESIAN_POINT('Ctrl Pts',(64.9503835492167,-7.85328451410953,-8.84701605985931));
#6351=CARTESIAN_POINT('Ctrl Pts',(64.9503835492166,-3.73732509952793,-11.2273777955275));
#6352=CARTESIAN_POINT('Ctrl Pts',(64.9503835492166,2.02072503306777,-11.6578836833029));
#6353=CARTESIAN_POINT('Ctrl Pts',(64.9503835492167,7.0051562897937,-9.7061677097367));
#6354=CARTESIAN_POINT('Ctrl Pts',(64.9503835492166,10.6478183083747,-5.12258043111314));
#6355=CARTESIAN_POINT('Ctrl Pts',(64.9503835492167,11.4278882091416,-1.70953167870107));
#6356=CARTESIAN_POINT('Ctrl Pts',(64.9503835492167,11.4278882091416,-4.57627715103496E-16));
#6357=CARTESIAN_POINT('',(64.9503835492166,11.4278882091416,1.38777878078145E-16));
#6358=CARTESIAN_POINT('Origin',(65.4451561127438,11.5,-5.55111512312578E-16));
#6359=CARTESIAN_POINT('Ctrl Pts',(64.9503835492167,11.4278882091416,-4.57627715103496E-16));
#6360=CARTESIAN_POINT('Ctrl Pts',(64.9503835492167,11.4278882091416,-1.70953167870107));
#6361=CARTESIAN_POINT('Ctrl Pts',(64.9503835492166,10.6478183083747,-5.12258043111314));
#6362=CARTESIAN_POINT('Ctrl Pts',(64.9503835492167,7.0051562897937,-9.7061677097367));
#6363=CARTESIAN_POINT('Ctrl Pts',(64.9503835492166,2.02072503306777,-11.6578836833029));
#6364=CARTESIAN_POINT('Ctrl Pts',(64.9503835492166,-3.73732509952793,-11.2273777955275));
#6365=CARTESIAN_POINT('Ctrl Pts',(64.9503835492167,-7.85328451410953,-8.84701605985931));
#6366=CARTESIAN_POINT('Ctrl Pts',(64.9503835492166,-11.1049444308876,-4.0790349306743));
#6367=CARTESIAN_POINT('Ctrl Pts',(64.9503835492166,-11.8197602196346,0.6260287266476));
#6368=CARTESIAN_POINT('Ctrl Pts',(64.9503835492167,-10.4470164004438,5.03171767144541));
#6369=CARTESIAN_POINT('Ctrl Pts',(64.9503835492167,-7.86014113917398,8.84867250689127));
#6370=CARTESIAN_POINT('Ctrl Pts',(64.9503835492166,-3.21708112269002,11.5281558506245));
#6371=CARTESIAN_POINT('Ctrl Pts',(64.9503835492167,2.63092921137885,11.519592989277));
#6372=CARTESIAN_POINT('Ctrl Pts',(64.9503835492166,7.36797152942324,9.24151515780478));
#6373=CARTESIAN_POINT('Ctrl Pts',(64.9503835492166,10.6485396706842,5.12709861319939));
#6374=CARTESIAN_POINT('Ctrl Pts',(64.9503835492166,11.4278882091416,1.70953167870107));
#6375=CARTESIAN_POINT('Ctrl Pts',(64.9503835492166,11.4278882091416,-5.94987561328448E-16));
#6376=CARTESIAN_POINT('Ctrl Pts',(58.1,25.5,0.));
#6377=CARTESIAN_POINT('Ctrl Pts',(58.1,25.5,25.5));
#6378=CARTESIAN_POINT('Ctrl Pts',(58.1,0.,25.5));
#6379=CARTESIAN_POINT('Ctrl Pts',(58.1,-25.5,25.5));
#6380=CARTESIAN_POINT('Ctrl Pts',(58.1,-25.5,0.));
#6381=CARTESIAN_POINT('Ctrl Pts',(58.1,-25.5,-25.5));
#6382=CARTESIAN_POINT('Ctrl Pts',(58.1,0.,-25.5));
#6383=CARTESIAN_POINT('Ctrl Pts',(58.1,25.5,-25.5));
#6384=CARTESIAN_POINT('Ctrl Pts',(58.1,25.5,0.));
#6385=CARTESIAN_POINT('Ctrl Pts',(58.1006850861903,25.3693230990265,0.));
#6386=CARTESIAN_POINT('Ctrl Pts',(58.1006850861903,25.3693230990265,25.3693230990265));
#6387=CARTESIAN_POINT('Ctrl Pts',(58.1006850861903,0.,25.3693230990265));
#6388=CARTESIAN_POINT('Ctrl Pts',(58.1006850861903,-25.3693230990265,25.3693230990265));
#6389=CARTESIAN_POINT('Ctrl Pts',(58.1006850861903,-25.3693230990265,0.));
#6390=CARTESIAN_POINT('Ctrl Pts',(58.1006850861903,-25.3693230990265,-25.3693230990265));
#6391=CARTESIAN_POINT('Ctrl Pts',(58.1006850861903,0.,-25.3693230990265));
#6392=CARTESIAN_POINT('Ctrl Pts',(58.1006850861903,25.3693230990265,-25.3693230990265));
#6393=CARTESIAN_POINT('Ctrl Pts',(58.1006850861903,25.3693230990265,0.));
#6394=CARTESIAN_POINT('Ctrl Pts',(58.106842887577,25.1090017061965,0.));
#6395=CARTESIAN_POINT('Ctrl Pts',(58.106842887577,25.1090017061965,25.1090017061965));
#6396=CARTESIAN_POINT('Ctrl Pts',(58.106842887577,0.,25.1090017061965));
#6397=CARTESIAN_POINT('Ctrl Pts',(58.106842887577,-25.1090017061965,25.1090017061965));
#6398=CARTESIAN_POINT('Ctrl Pts',(58.106842887577,-25.1090017061965,0.));
#6399=CARTESIAN_POINT('Ctrl Pts',(58.106842887577,-25.1090017061965,-25.1090017061965));
#6400=CARTESIAN_POINT('Ctrl Pts',(58.106842887577,0.,-25.1090017061965));
#6401=CARTESIAN_POINT('Ctrl Pts',(58.106842887577,25.1090017061965,-25.1090017061965));
#6402=CARTESIAN_POINT('Ctrl Pts',(58.106842887577,25.1090017061965,0.));
#6403=CARTESIAN_POINT('Ctrl Pts',(58.1304424850882,24.7216168481987,0.));
#6404=CARTESIAN_POINT('Ctrl Pts',(58.1304424850882,24.7216168481987,24.7216168481987));
#6405=CARTESIAN_POINT('Ctrl Pts',(58.1304424850882,0.,24.7216168481987));
#6406=CARTESIAN_POINT('Ctrl Pts',(58.1304424850882,-24.7216168481987,24.7216168481987));
#6407=CARTESIAN_POINT('Ctrl Pts',(58.1304424850882,-24.7216168481987,0.));
#6408=CARTESIAN_POINT('Ctrl Pts',(58.1304424850882,-24.7216168481987,-24.7216168481987));
#6409=CARTESIAN_POINT('Ctrl Pts',(58.1304424850882,0.,-24.7216168481987));
#6410=CARTESIAN_POINT('Ctrl Pts',(58.1304424850882,24.7216168481987,-24.7216168481987));
#6411=CARTESIAN_POINT('Ctrl Pts',(58.1304424850882,24.7216168481987,0.));
#6412=CARTESIAN_POINT('Ctrl Pts',(58.1907092774481,24.2113142943935,0.));
#6413=CARTESIAN_POINT('Ctrl Pts',(58.1907092774481,24.2113142943935,24.2113142943935));
#6414=CARTESIAN_POINT('Ctrl Pts',(58.1907092774481,0.,24.2113142943935));
#6415=CARTESIAN_POINT('Ctrl Pts',(58.1907092774481,-24.2113142943935,24.2113142943935));
#6416=CARTESIAN_POINT('Ctrl Pts',(58.1907092774481,-24.2113142943935,0.));
#6417=CARTESIAN_POINT('Ctrl Pts',(58.1907092774481,-24.2113142943935,-24.2113142943935));
#6418=CARTESIAN_POINT('Ctrl Pts',(58.1907092774481,0.,-24.2113142943935));
#6419=CARTESIAN_POINT('Ctrl Pts',(58.1907092774481,24.2113142943935,-24.2113142943935));
#6420=CARTESIAN_POINT('Ctrl Pts',(58.1907092774481,24.2113142943935,0.));
#6421=CARTESIAN_POINT('Ctrl Pts',(58.3142240203109,23.5838111702086,0.));
#6422=CARTESIAN_POINT('Ctrl Pts',(58.3142240203109,23.5838111702086,23.5838111702086));
#6423=CARTESIAN_POINT('Ctrl Pts',(58.3142240203109,0.,23.5838111702086));
#6424=CARTESIAN_POINT('Ctrl Pts',(58.3142240203109,-23.5838111702086,23.5838111702086));
#6425=CARTESIAN_POINT('Ctrl Pts',(58.3142240203109,-23.5838111702086,0.));
#6426=CARTESIAN_POINT('Ctrl Pts',(58.3142240203109,-23.5838111702086,-23.5838111702086));
#6427=CARTESIAN_POINT('Ctrl Pts',(58.3142240203109,0.,-23.5838111702086));
#6428=CARTESIAN_POINT('Ctrl Pts',(58.3142240203109,23.5838111702086,-23.5838111702086));
#6429=CARTESIAN_POINT('Ctrl Pts',(58.3142240203109,23.5838111702086,0.));
#6430=CARTESIAN_POINT('Ctrl Pts',(58.4856917608691,22.9665891529976,0.));
#6431=CARTESIAN_POINT('Ctrl Pts',(58.4856917608691,22.9665891529976,22.9665891529976));
#6432=CARTESIAN_POINT('Ctrl Pts',(58.4856917608691,0.,22.9665891529976));
#6433=CARTESIAN_POINT('Ctrl Pts',(58.4856917608691,-22.9665891529976,22.9665891529976));
#6434=CARTESIAN_POINT('Ctrl Pts',(58.4856917608691,-22.9665891529976,0.));
#6435=CARTESIAN_POINT('Ctrl Pts',(58.4856917608691,-22.9665891529976,-22.9665891529976));
#6436=CARTESIAN_POINT('Ctrl Pts',(58.4856917608691,0.,-22.9665891529976));
#6437=CARTESIAN_POINT('Ctrl Pts',(58.4856917608691,22.9665891529976,-22.9665891529976));
#6438=CARTESIAN_POINT('Ctrl Pts',(58.4856917608691,22.9665891529976,0.));
#6439=CARTESIAN_POINT('Ctrl Pts',(58.7040649536582,22.3593331170216,0.));
#6440=CARTESIAN_POINT('Ctrl Pts',(58.7040649536582,22.3593331170216,22.3593331170216));
#6441=CARTESIAN_POINT('Ctrl Pts',(58.7040649536582,0.,22.3593331170216));
#6442=CARTESIAN_POINT('Ctrl Pts',(58.7040649536582,-22.3593331170216,22.3593331170216));
#6443=CARTESIAN_POINT('Ctrl Pts',(58.7040649536582,-22.3593331170216,0.));
#6444=CARTESIAN_POINT('Ctrl Pts',(58.7040649536582,-22.3593331170216,-22.3593331170216));
#6445=CARTESIAN_POINT('Ctrl Pts',(58.7040649536582,0.,-22.3593331170216));
#6446=CARTESIAN_POINT('Ctrl Pts',(58.7040649536582,22.3593331170216,-22.3593331170216));
#6447=CARTESIAN_POINT('Ctrl Pts',(58.7040649536582,22.3593331170216,0.));
#6448=CARTESIAN_POINT('Ctrl Pts',(58.9670233800433,21.7613919711372,0.));
#6449=CARTESIAN_POINT('Ctrl Pts',(58.9670233800433,21.7613919711372,21.7613919711372));
#6450=CARTESIAN_POINT('Ctrl Pts',(58.9670233800433,0.,21.7613919711372));
#6451=CARTESIAN_POINT('Ctrl Pts',(58.9670233800433,-21.7613919711372,21.7613919711372));
#6452=CARTESIAN_POINT('Ctrl Pts',(58.9670233800433,-21.7613919711372,0.));
#6453=CARTESIAN_POINT('Ctrl Pts',(58.9670233800433,-21.7613919711372,-21.7613919711372));
#6454=CARTESIAN_POINT('Ctrl Pts',(58.9670233800433,0.,-21.7613919711372));
#6455=CARTESIAN_POINT('Ctrl Pts',(58.9670233800433,21.7613919711372,-21.7613919711372));
#6456=CARTESIAN_POINT('Ctrl Pts',(58.9670233800433,21.7613919711372,0.));
#6457=CARTESIAN_POINT('Ctrl Pts',(59.2705528391893,21.1716763589853,0.));
#6458=CARTESIAN_POINT('Ctrl Pts',(59.2705528391893,21.1716763589853,21.1716763589853));
#6459=CARTESIAN_POINT('Ctrl Pts',(59.2705528391893,0.,21.1716763589853));
#6460=CARTESIAN_POINT('Ctrl Pts',(59.2705528391893,-21.1716763589853,21.1716763589853));
#6461=CARTESIAN_POINT('Ctrl Pts',(59.2705528391893,-21.1716763589853,0.));
#6462=CARTESIAN_POINT('Ctrl Pts',(59.2705528391893,-21.1716763589853,-21.1716763589853));
#6463=CARTESIAN_POINT('Ctrl Pts',(59.2705528391893,0.,-21.1716763589853));
#6464=CARTESIAN_POINT('Ctrl Pts',(59.2705528391893,21.1716763589853,-21.1716763589853));
#6465=CARTESIAN_POINT('Ctrl Pts',(59.2705528391893,21.1716763589853,0.));
#6466=CARTESIAN_POINT('Ctrl Pts',(59.6094227136446,20.5888495299376,0.));
#6467=CARTESIAN_POINT('Ctrl Pts',(59.6094227136446,20.5888495299376,20.5888495299376));
#6468=CARTESIAN_POINT('Ctrl Pts',(59.6094227136446,0.,20.5888495299376));
#6469=CARTESIAN_POINT('Ctrl Pts',(59.6094227136446,-20.5888495299376,20.5888495299376));
#6470=CARTESIAN_POINT('Ctrl Pts',(59.6094227136446,-20.5888495299376,0.));
#6471=CARTESIAN_POINT('Ctrl Pts',(59.6094227136446,-20.5888495299376,-20.5888495299376));
#6472=CARTESIAN_POINT('Ctrl Pts',(59.6094227136446,0.,-20.5888495299376));
#6473=CARTESIAN_POINT('Ctrl Pts',(59.6094227136446,20.5888495299376,-20.5888495299376));
#6474=CARTESIAN_POINT('Ctrl Pts',(59.6094227136446,20.5888495299376,0.));
#6475=CARTESIAN_POINT('Ctrl Pts',(59.9775897880897,20.0114964775053,0.));
#6476=CARTESIAN_POINT('Ctrl Pts',(59.9775897880897,20.0114964775053,20.0114964775053));
#6477=CARTESIAN_POINT('Ctrl Pts',(59.9775897880897,0.,20.0114964775053));
#6478=CARTESIAN_POINT('Ctrl Pts',(59.9775897880897,-20.0114964775053,20.0114964775053));
#6479=CARTESIAN_POINT('Ctrl Pts',(59.9775897880897,-20.0114964775053,0.));
#6480=CARTESIAN_POINT('Ctrl Pts',(59.9775897880897,-20.0114964775053,-20.0114964775053));
#6481=CARTESIAN_POINT('Ctrl Pts',(59.9775897880897,0.,-20.0114964775053));
#6482=CARTESIAN_POINT('Ctrl Pts',(59.9775897880897,20.0114964775053,-20.0114964775053));
#6483=CARTESIAN_POINT('Ctrl Pts',(59.9775897880897,20.0114964775053,0.));
#6484=CARTESIAN_POINT('Ctrl Pts',(60.3686078898803,19.4382992332324,0.));
#6485=CARTESIAN_POINT('Ctrl Pts',(60.3686078898803,19.4382992332324,19.4382992332324));
#6486=CARTESIAN_POINT('Ctrl Pts',(60.3686078898803,0.,19.4382992332324));
#6487=CARTESIAN_POINT('Ctrl Pts',(60.3686078898803,-19.4382992332324,19.4382992332324));
#6488=CARTESIAN_POINT('Ctrl Pts',(60.3686078898803,-19.4382992332324,0.));
#6489=CARTESIAN_POINT('Ctrl Pts',(60.3686078898803,-19.4382992332324,-19.4382992332324));
#6490=CARTESIAN_POINT('Ctrl Pts',(60.3686078898803,0.,-19.4382992332324));
#6491=CARTESIAN_POINT('Ctrl Pts',(60.3686078898803,19.4382992332324,-19.4382992332324));
#6492=CARTESIAN_POINT('Ctrl Pts',(60.3686078898803,19.4382992332324,0.));
#6493=CARTESIAN_POINT('Ctrl Pts',(60.7760056975964,18.8682016392444,0.));
#6494=CARTESIAN_POINT('Ctrl Pts',(60.7760056975964,18.8682016392444,18.8682016392444));
#6495=CARTESIAN_POINT('Ctrl Pts',(60.7760056975964,0.,18.8682016392444));
#6496=CARTESIAN_POINT('Ctrl Pts',(60.7760056975964,-18.8682016392444,18.8682016392444));
#6497=CARTESIAN_POINT('Ctrl Pts',(60.7760056975964,-18.8682016392444,0.));
#6498=CARTESIAN_POINT('Ctrl Pts',(60.7760056975964,-18.8682016392444,-18.8682016392444));
#6499=CARTESIAN_POINT('Ctrl Pts',(60.7760056975964,0.,-18.8682016392444));
#6500=CARTESIAN_POINT('Ctrl Pts',(60.7760056975964,18.8682016392444,-18.8682016392444));
#6501=CARTESIAN_POINT('Ctrl Pts',(60.7760056975964,18.8682016392444,0.));
#6502=CARTESIAN_POINT('Ctrl Pts',(61.1936904784186,18.3005942681782,0.));
#6503=CARTESIAN_POINT('Ctrl Pts',(61.1936904784186,18.3005942681782,18.3005942681782));
#6504=CARTESIAN_POINT('Ctrl Pts',(61.1936904784186,0.,18.3005942681782));
#6505=CARTESIAN_POINT('Ctrl Pts',(61.1936904784186,-18.3005942681782,18.3005942681782));
#6506=CARTESIAN_POINT('Ctrl Pts',(61.1936904784186,-18.3005942681782,0.));
#6507=CARTESIAN_POINT('Ctrl Pts',(61.1936904784186,-18.3005942681782,-18.3005942681782));
#6508=CARTESIAN_POINT('Ctrl Pts',(61.1936904784186,0.,-18.3005942681782));
#6509=CARTESIAN_POINT('Ctrl Pts',(61.1936904784186,18.3005942681782,-18.3005942681782));
#6510=CARTESIAN_POINT('Ctrl Pts',(61.1936904784186,18.3005942681782,0.));
#6511=CARTESIAN_POINT('Ctrl Pts',(61.6158386260792,17.7351881055358,0.));
#6512=CARTESIAN_POINT('Ctrl Pts',(61.6158386260792,17.7351881055358,17.7351881055358));
#6513=CARTESIAN_POINT('Ctrl Pts',(61.6158386260792,0.,17.7351881055358));
#6514=CARTESIAN_POINT('Ctrl Pts',(61.6158386260792,-17.7351881055358,17.7351881055358));
#6515=CARTESIAN_POINT('Ctrl Pts',(61.6158386260792,-17.7351881055358,0.));
#6516=CARTESIAN_POINT('Ctrl Pts',(61.6158386260792,-17.7351881055358,-17.7351881055358));
#6517=CARTESIAN_POINT('Ctrl Pts',(61.6158386260792,0.,-17.7351881055358));
#6518=CARTESIAN_POINT('Ctrl Pts',(61.6158386260792,17.7351881055358,-17.7351881055358));
#6519=CARTESIAN_POINT('Ctrl Pts',(61.6158386260792,17.7351881055358,0.));
#6520=CARTESIAN_POINT('Ctrl Pts',(62.0367583558289,17.1718725504246,0.));
#6521=CARTESIAN_POINT('Ctrl Pts',(62.0367583558289,17.1718725504246,17.1718725504246));
#6522=CARTESIAN_POINT('Ctrl Pts',(62.0367583558289,0.,17.1718725504246));
#6523=CARTESIAN_POINT('Ctrl Pts',(62.0367583558289,-17.1718725504246,17.1718725504246));
#6524=CARTESIAN_POINT('Ctrl Pts',(62.0367583558289,-17.1718725504246,0.));
#6525=CARTESIAN_POINT('Ctrl Pts',(62.0367583558289,-17.1718725504246,-17.1718725504246));
#6526=CARTESIAN_POINT('Ctrl Pts',(62.0367583558289,0.,-17.1718725504246));
#6527=CARTESIAN_POINT('Ctrl Pts',(62.0367583558289,17.1718725504246,-17.1718725504246));
#6528=CARTESIAN_POINT('Ctrl Pts',(62.0367583558289,17.1718725504246,0.));
#6529=CARTESIAN_POINT('Ctrl Pts',(62.4507485326533,16.6105738821721,0.));
#6530=CARTESIAN_POINT('Ctrl Pts',(62.4507485326533,16.6105738821721,16.6105738821721));
#6531=CARTESIAN_POINT('Ctrl Pts',(62.4507485326533,0.,16.6105738821721));
#6532=CARTESIAN_POINT('Ctrl Pts',(62.4507485326533,-16.6105738821721,16.6105738821721));
#6533=CARTESIAN_POINT('Ctrl Pts',(62.4507485326533,-16.6105738821721,0.));
#6534=CARTESIAN_POINT('Ctrl Pts',(62.4507485326533,-16.6105738821721,-16.6105738821721));
#6535=CARTESIAN_POINT('Ctrl Pts',(62.4507485326533,0.,-16.6105738821721));
#6536=CARTESIAN_POINT('Ctrl Pts',(62.4507485326533,16.6105738821721,-16.6105738821721));
#6537=CARTESIAN_POINT('Ctrl Pts',(62.4507485326533,16.6105738821721,0.));
#6538=CARTESIAN_POINT('Ctrl Pts',(62.8519889360609,16.0511281710465,0.));
#6539=CARTESIAN_POINT('Ctrl Pts',(62.8519889360609,16.0511281710465,16.0511281710465));
#6540=CARTESIAN_POINT('Ctrl Pts',(62.8519889360609,0.,16.0511281710465));
#6541=CARTESIAN_POINT('Ctrl Pts',(62.8519889360609,-16.0511281710465,16.0511281710465));
#6542=CARTESIAN_POINT('Ctrl Pts',(62.8519889360609,-16.0511281710465,0.));
#6543=CARTESIAN_POINT('Ctrl Pts',(62.8519889360609,-16.0511281710465,-16.0511281710465));
#6544=CARTESIAN_POINT('Ctrl Pts',(62.8519889360609,0.,-16.0511281710465));
#6545=CARTESIAN_POINT('Ctrl Pts',(62.8519889360609,16.0511281710465,-16.0511281710465));
#6546=CARTESIAN_POINT('Ctrl Pts',(62.8519889360609,16.0511281710465,0.));
#6547=CARTESIAN_POINT('Ctrl Pts',(63.2343441839831,15.4931095154543,0.));
#6548=CARTESIAN_POINT('Ctrl Pts',(63.2343441839831,15.4931095154543,15.4931095154543));
#6549=CARTESIAN_POINT('Ctrl Pts',(63.2343441839831,0.,15.4931095154543));
#6550=CARTESIAN_POINT('Ctrl Pts',(63.2343441839831,-15.4931095154543,15.4931095154543));
#6551=CARTESIAN_POINT('Ctrl Pts',(63.2343441839831,-15.4931095154543,0.));
#6552=CARTESIAN_POINT('Ctrl Pts',(63.2343441839831,-15.4931095154543,-15.4931095154543));
#6553=CARTESIAN_POINT('Ctrl Pts',(63.2343441839831,0.,-15.4931095154543));
#6554=CARTESIAN_POINT('Ctrl Pts',(63.2343441839831,15.4931095154543,-15.4931095154543));
#6555=CARTESIAN_POINT('Ctrl Pts',(63.2343441839831,15.4931095154543,0.));
#6556=CARTESIAN_POINT('Ctrl Pts',(63.5915578634715,14.9358503082954,0.));
#6557=CARTESIAN_POINT('Ctrl Pts',(63.5915578634715,14.9358503082954,14.9358503082954));
#6558=CARTESIAN_POINT('Ctrl Pts',(63.5915578634715,0.,14.9358503082954));
#6559=CARTESIAN_POINT('Ctrl Pts',(63.5915578634715,-14.9358503082954,14.9358503082954));
#6560=CARTESIAN_POINT('Ctrl Pts',(63.5915578634715,-14.9358503082954,0.));
#6561=CARTESIAN_POINT('Ctrl Pts',(63.5915578634715,-14.9358503082954,-14.9358503082954));
#6562=CARTESIAN_POINT('Ctrl Pts',(63.5915578634715,0.,-14.9358503082954));
#6563=CARTESIAN_POINT('Ctrl Pts',(63.5915578634715,14.9358503082954,-14.9358503082954));
#6564=CARTESIAN_POINT('Ctrl Pts',(63.5915578634715,14.9358503082954,0.));
#6565=CARTESIAN_POINT('Ctrl Pts',(63.9176667121215,14.3785717762628,0.));
#6566=CARTESIAN_POINT('Ctrl Pts',(63.9176667121215,14.3785717762628,14.3785717762628));
#6567=CARTESIAN_POINT('Ctrl Pts',(63.9176667121215,0.,14.3785717762628));
#6568=CARTESIAN_POINT('Ctrl Pts',(63.9176667121215,-14.3785717762628,14.3785717762628));
#6569=CARTESIAN_POINT('Ctrl Pts',(63.9176667121215,-14.3785717762628,0.));
#6570=CARTESIAN_POINT('Ctrl Pts',(63.9176667121215,-14.3785717762628,-14.3785717762628));
#6571=CARTESIAN_POINT('Ctrl Pts',(63.9176667121215,0.,-14.3785717762628));
#6572=CARTESIAN_POINT('Ctrl Pts',(63.9176667121215,14.3785717762628,-14.3785717762628));
#6573=CARTESIAN_POINT('Ctrl Pts',(63.9176667121215,14.3785717762628,0.));
#6574=CARTESIAN_POINT('Ctrl Pts',(64.2073839217625,13.8204835129561,0.));
#6575=CARTESIAN_POINT('Ctrl Pts',(64.2073839217625,13.8204835129561,13.8204835129561));
#6576=CARTESIAN_POINT('Ctrl Pts',(64.2073839217625,0.,13.8204835129561));
#6577=CARTESIAN_POINT('Ctrl Pts',(64.2073839217625,-13.8204835129561,13.8204835129561));
#6578=CARTESIAN_POINT('Ctrl Pts',(64.2073839217625,-13.8204835129561,0.));
#6579=CARTESIAN_POINT('Ctrl Pts',(64.2073839217625,-13.8204835129561,-13.8204835129561));
#6580=CARTESIAN_POINT('Ctrl Pts',(64.2073839217625,0.,-13.8204835129561));
#6581=CARTESIAN_POINT('Ctrl Pts',(64.2073839217625,13.8204835129561,-13.8204835129561));
#6582=CARTESIAN_POINT('Ctrl Pts',(64.2073839217625,13.8204835129561,0.));
#6583=CARTESIAN_POINT('Ctrl Pts',(64.4564605946371,13.2608853560062,0.));
#6584=CARTESIAN_POINT('Ctrl Pts',(64.4564605946371,13.2608853560062,13.2608853560062));
#6585=CARTESIAN_POINT('Ctrl Pts',(64.4564605946371,0.,13.2608853560062));
#6586=CARTESIAN_POINT('Ctrl Pts',(64.4564605946371,-13.2608853560062,13.2608853560062));
#6587=CARTESIAN_POINT('Ctrl Pts',(64.4564605946371,-13.2608853560062,0.));
#6588=CARTESIAN_POINT('Ctrl Pts',(64.4564605946371,-13.2608853560062,-13.2608853560062));
#6589=CARTESIAN_POINT('Ctrl Pts',(64.4564605946371,0.,-13.2608853560062));
#6590=CARTESIAN_POINT('Ctrl Pts',(64.4564605946371,13.2608853560062,-13.2608853560062));
#6591=CARTESIAN_POINT('Ctrl Pts',(64.4564605946371,13.2608853560062,0.));
#6592=CARTESIAN_POINT('Ctrl Pts',(64.6622177060836,12.6992939860082,0.));
#6593=CARTESIAN_POINT('Ctrl Pts',(64.6622177060836,12.6992939860082,12.6992939860082));
#6594=CARTESIAN_POINT('Ctrl Pts',(64.6622177060836,0.,12.6992939860082));
#6595=CARTESIAN_POINT('Ctrl Pts',(64.6622177060836,-12.6992939860082,12.6992939860082));
#6596=CARTESIAN_POINT('Ctrl Pts',(64.6622177060836,-12.6992939860082,0.));
#6597=CARTESIAN_POINT('Ctrl Pts',(64.6622177060836,-12.6992939860082,-12.6992939860082));
#6598=CARTESIAN_POINT('Ctrl Pts',(64.6622177060836,0.,-12.6992939860082));
#6599=CARTESIAN_POINT('Ctrl Pts',(64.6622177060836,12.6992939860082,-12.6992939860082));
#6600=CARTESIAN_POINT('Ctrl Pts',(64.6622177060836,12.6992939860082,0.));
#6601=CARTESIAN_POINT('Ctrl Pts',(64.8234125059507,12.1354463894458,0.));
#6602=CARTESIAN_POINT('Ctrl Pts',(64.8234125059507,12.1354463894458,12.1354463894458));
#6603=CARTESIAN_POINT('Ctrl Pts',(64.8234125059507,0.,12.1354463894458));
#6604=CARTESIAN_POINT('Ctrl Pts',(64.8234125059507,-12.1354463894458,12.1354463894458));
#6605=CARTESIAN_POINT('Ctrl Pts',(64.8234125059507,-12.1354463894458,0.));
#6606=CARTESIAN_POINT('Ctrl Pts',(64.8234125059507,-12.1354463894458,-12.1354463894458));
#6607=CARTESIAN_POINT('Ctrl Pts',(64.8234125059507,0.,-12.1354463894458));
#6608=CARTESIAN_POINT('Ctrl Pts',(64.8234125059507,12.1354463894458,-12.1354463894458));
#6609=CARTESIAN_POINT('Ctrl Pts',(64.8234125059507,12.1354463894458,0.));
#6610=CARTESIAN_POINT('Ctrl Pts',(64.916430253722,11.6824677271476,0.));
#6611=CARTESIAN_POINT('Ctrl Pts',(64.916430253722,11.6824677271476,11.6824677271476));
#6612=CARTESIAN_POINT('Ctrl Pts',(64.916430253722,0.,11.6824677271476));
#6613=CARTESIAN_POINT('Ctrl Pts',(64.916430253722,-11.6824677271476,11.6824677271476));
#6614=CARTESIAN_POINT('Ctrl Pts',(64.916430253722,-11.6824677271476,0.));
#6615=CARTESIAN_POINT('Ctrl Pts',(64.916430253722,-11.6824677271476,-11.6824677271476));
#6616=CARTESIAN_POINT('Ctrl Pts',(64.916430253722,0.,-11.6824677271476));
#6617=CARTESIAN_POINT('Ctrl Pts',(64.916430253722,11.6824677271476,-11.6824677271476));
#6618=CARTESIAN_POINT('Ctrl Pts',(64.916430253722,11.6824677271476,0.));
#6619=CARTESIAN_POINT('Ctrl Pts',(64.9660346030933,11.3416530788372,0.));
#6620=CARTESIAN_POINT('Ctrl Pts',(64.9660346030933,11.3416530788372,11.3416530788372));
#6621=CARTESIAN_POINT('Ctrl Pts',(64.9660346030933,0.,11.3416530788372));
#6622=CARTESIAN_POINT('Ctrl Pts',(64.9660346030933,-11.3416530788372,11.3416530788372));
#6623=CARTESIAN_POINT('Ctrl Pts',(64.9660346030933,-11.3416530788372,0.));
#6624=CARTESIAN_POINT('Ctrl Pts',(64.9660346030933,-11.3416530788372,-11.3416530788372));
#6625=CARTESIAN_POINT('Ctrl Pts',(64.9660346030933,0.,-11.3416530788372));
#6626=CARTESIAN_POINT('Ctrl Pts',(64.9660346030933,11.3416530788372,-11.3416530788372));
#6627=CARTESIAN_POINT('Ctrl Pts',(64.9660346030933,11.3416530788372,0.));
#6628=CARTESIAN_POINT('Ctrl Pts',(64.9901676141296,11.1139642079645,0.));
#6629=CARTESIAN_POINT('Ctrl Pts',(64.9901676141296,11.1139642079645,11.1139642079645));
#6630=CARTESIAN_POINT('Ctrl Pts',(64.9901676141296,0.,11.1139642079645));
#6631=CARTESIAN_POINT('Ctrl Pts',(64.9901676141296,-11.1139642079645,11.1139642079645));
#6632=CARTESIAN_POINT('Ctrl Pts',(64.9901676141296,-11.1139642079645,0.));
#6633=CARTESIAN_POINT('Ctrl Pts',(64.9901676141296,-11.1139642079645,-11.1139642079645));
#6634=CARTESIAN_POINT('Ctrl Pts',(64.9901676141296,0.,-11.1139642079645));
#6635=CARTESIAN_POINT('Ctrl Pts',(64.9901676141296,11.1139642079645,-11.1139642079645));
#6636=CARTESIAN_POINT('Ctrl Pts',(64.9901676141296,11.1139642079645,0.));
#6637=CARTESIAN_POINT('Ctrl Pts',(65.,11.,0.));
#6638=CARTESIAN_POINT('Ctrl Pts',(65.,11.,11.));
#6639=CARTESIAN_POINT('Ctrl Pts',(65.,0.,11.));
#6640=CARTESIAN_POINT('Ctrl Pts',(65.,-11.,11.));
#6641=CARTESIAN_POINT('Ctrl Pts',(65.,-11.,0.));
#6642=CARTESIAN_POINT('Ctrl Pts',(65.,-11.,-11.));
#6643=CARTESIAN_POINT('Ctrl Pts',(65.,0.,-11.));
#6644=CARTESIAN_POINT('Ctrl Pts',(65.,11.,-11.));
#6645=CARTESIAN_POINT('Ctrl Pts',(65.,11.,0.));
#6646=CARTESIAN_POINT('',(58.1000072797208,25.4986314827274,3.83026943495679E-14));
#6647=CARTESIAN_POINT('Ctrl Pts',(58.1000072797208,25.4986314827274,0.));
#6648=CARTESIAN_POINT('Ctrl Pts',(58.1007109447233,25.3682326055233,0.));
#6649=CARTESIAN_POINT('Ctrl Pts',(58.1068923494636,25.1081903199643,0.));
#6650=CARTESIAN_POINT('Ctrl Pts',(58.1305056112578,24.7210824259432,0.));
#6651=CARTESIAN_POINT('Ctrl Pts',(58.1907610187597,24.2110514283266,0.));
#6652=CARTESIAN_POINT('Ctrl Pts',(58.3142240203109,23.5838111702086,0.));
#6653=CARTESIAN_POINT('Ctrl Pts',(58.4856917608691,22.9665891529976,0.));
#6654=CARTESIAN_POINT('Ctrl Pts',(58.7040649536582,22.3593331170216,0.));
#6655=CARTESIAN_POINT('Ctrl Pts',(58.9670233800433,21.7613919711372,0.));
#6656=CARTESIAN_POINT('Ctrl Pts',(59.2705528391893,21.1716763589853,0.));
#6657=CARTESIAN_POINT('Ctrl Pts',(59.6094227136446,20.5888495299376,0.));
#6658=CARTESIAN_POINT('Ctrl Pts',(59.9775897880897,20.0114964775053,0.));
#6659=CARTESIAN_POINT('Ctrl Pts',(60.3686078898803,19.4382992332324,0.));
#6660=CARTESIAN_POINT('Ctrl Pts',(60.7760056975964,18.8682016392444,0.));
#6661=CARTESIAN_POINT('Ctrl Pts',(61.1936904784186,18.3005942681782,0.));
#6662=CARTESIAN_POINT('Ctrl Pts',(61.6158386260792,17.7351881055358,0.));
#6663=CARTESIAN_POINT('Ctrl Pts',(62.0367583558289,17.1718725504246,0.));
#6664=CARTESIAN_POINT('Ctrl Pts',(62.4507485326533,16.6105738821721,0.));
#6665=CARTESIAN_POINT('Ctrl Pts',(62.8519889360609,16.0511281710465,0.));
#6666=CARTESIAN_POINT('Ctrl Pts',(63.2343441839831,15.4931095154543,0.));
#6667=CARTESIAN_POINT('Ctrl Pts',(63.5915578634715,14.9358503082954,0.));
#6668=CARTESIAN_POINT('Ctrl Pts',(63.9176667121215,14.3785717762628,0.));
#6669=CARTESIAN_POINT('Ctrl Pts',(64.2073839217625,13.8204835129561,0.));
#6670=CARTESIAN_POINT('Ctrl Pts',(64.4564605946371,13.2608853560062,0.));
#6671=CARTESIAN_POINT('Ctrl Pts',(64.6622177060836,12.6992939860082,0.));
#6672=CARTESIAN_POINT('Ctrl Pts',(64.7991653885414,12.2202610291617,0.));
#6673=CARTESIAN_POINT('Ctrl Pts',(64.8801800932063,11.8527445341239,0.));
#6674=CARTESIAN_POINT('Ctrl Pts',(64.9249249220199,11.5977782643751,0.));
#6675=CARTESIAN_POINT('Ctrl Pts',(64.9462790584754,11.4560498922985,0.));
#6676=CARTESIAN_POINT('Ctrl Pts',(64.9503835492167,11.4278882091416,0.));
#6677=CARTESIAN_POINT('Ctrl Pts',(58.1000072797208,25.4986314827289,2.38697950294409E-14));
#6678=CARTESIAN_POINT('Ctrl Pts',(58.1000072797208,25.4986314827289,3.81441588205112));
#6679=CARTESIAN_POINT('Ctrl Pts',(58.1000072797208,23.7594464132255,11.4410395120049));
#6680=CARTESIAN_POINT('Ctrl Pts',(58.1000072797208,16.4420132235113,20.6165782938419));
#6681=CARTESIAN_POINT('Ctrl Pts',(58.1000072797208,5.8680831928706,25.709427795297));
#6682=CARTESIAN_POINT('Ctrl Pts',(58.1000072797208,-4.56335585676364,25.7079717649665));
#6683=CARTESIAN_POINT('Ctrl Pts',(58.1000072797208,-12.9396099811428,22.4138494830494));
#6684=CARTESIAN_POINT('Ctrl Pts',(58.1000072797208,-18.9752754976121,17.6048416816306));
#6685=CARTESIAN_POINT('Ctrl Pts',(58.1000072797208,-23.3123262403551,11.2305682370571));
#6686=CARTESIAN_POINT('Ctrl Pts',(58.1000072797208,-26.3703094632176,1.3980365463646));
#6687=CARTESIAN_POINT('Ctrl Pts',(58.1000072797208,-24.7834831225059,-9.10809204222051));
#6688=CARTESIAN_POINT('Ctrl Pts',(58.1000072797208,-18.9691368355184,-17.602615750836));
#6689=CARTESIAN_POINT('Ctrl Pts',(58.1000072797208,-12.9426554227937,-22.4171076785279));
#6690=CARTESIAN_POINT('Ctrl Pts',(58.1000072797208,-5.76030348627288,-25.2270747172432));
#6691=CARTESIAN_POINT('Ctrl Pts',(58.1000072797208,4.50410772030096,-26.0198514690206));
#6692=CARTESIAN_POINT('Ctrl Pts',(58.1000072797208,15.6329016549998,-21.6519940090828));
#6693=CARTESIAN_POINT('Ctrl Pts',(58.1000072797208,23.7567819506992,-11.4335435336754));
#6694=CARTESIAN_POINT('Ctrl Pts',(58.1000072797208,25.4986314827281,-3.81441588205099));
#6695=CARTESIAN_POINT('Ctrl Pts',(58.1000072797208,25.4986314827281,7.66053886991358E-14));
#6696=CARTESIAN_POINT('Origin',(66.5,0.,0.));
#6697=CARTESIAN_POINT('',(67.,-1.40834381901946E-15,11.5));
#6698=CARTESIAN_POINT('Origin',(66.5,-1.40834381901946E-15,11.5));
#6699=CARTESIAN_POINT('Origin',(67.,0.,0.));
#6700=CARTESIAN_POINT('Origin',(67.,11.,0.));
#6701=CARTESIAN_POINT('',(67.,12.5828687521281,-3.88578058618805E-15));
#6702=CARTESIAN_POINT('Ctrl Pts',(67.,12.5828687521281,-4.42954684098673E-15));
#6703=CARTESIAN_POINT('Ctrl Pts',(67.,12.5828687521281,-1.88230864242211));
#6704=CARTESIAN_POINT('Ctrl Pts',(67.,11.723903698598,-5.64071163506987));
#6705=CARTESIAN_POINT('Ctrl Pts',(67.,7.71284902408557,-10.6871388545133));
#6706=CARTESIAN_POINT('Ctrl Pts',(67.,2.22487832877622,-12.8362645212214));
#6707=CARTESIAN_POINT('Ctrl Pts',(67.,-4.11571491706988,-12.3615954421279));
#6708=CARTESIAN_POINT('Ctrl Pts',(67.,-8.6464168302479,-9.7416764263013));
#6709=CARTESIAN_POINT('Ctrl Pts',(67.,-12.2290791603529,-4.48959736793348));
#6710=CARTESIAN_POINT('Ctrl Pts',(67.,-13.010200205145,0.686125352829048));
#6711=CARTESIAN_POINT('Ctrl Pts',(67.,-11.1355356277156,6.76267604165808));
#6712=CARTESIAN_POINT('Ctrl Pts',(67.,-7.57288094607568,10.6000612069797));
#6713=CARTESIAN_POINT('Ctrl Pts',(67.,-2.24885032695964,12.6844091193373));
#6714=CARTESIAN_POINT('Ctrl Pts',(67.,2.89442276640883,12.6874499975273));
#6715=CARTESIAN_POINT('Ctrl Pts',(67.,8.11457746630642,10.1730735192044));
#6716=CARTESIAN_POINT('Ctrl Pts',(67.,11.7240714096075,5.64603610965329));
#6717=CARTESIAN_POINT('Ctrl Pts',(67.,12.5828687521281,1.8823086424221));
#6718=CARTESIAN_POINT('Ctrl Pts',(67.,12.5828687521281,8.21727726654077E-16));
#6719=CARTESIAN_POINT('Ctrl Pts',(66.9987790562313,12.6177894202923,8.32667268468867E-16));
#6720=CARTESIAN_POINT('Ctrl Pts',(66.9987790562313,12.6177894202923,1.88753252870585));
#6721=CARTESIAN_POINT('Ctrl Pts',(66.9987790562313,11.7566086962385,5.66170529903387));
#6722=CARTESIAN_POINT('Ctrl Pts',(66.9987790562313,8.13709748718362,10.2013063913397));
#6723=CARTESIAN_POINT('Ctrl Pts',(66.9987790562312,2.90245552737485,12.7226609053052));
#6724=CARTESIAN_POINT('Ctrl Pts',(66.9987790562313,-2.25509145984958,12.7196115879031));
#6725=CARTESIAN_POINT('Ctrl Pts',(66.9987790562313,-7.59389762103065,10.6294790787878));
#6726=CARTESIAN_POINT('Ctrl Pts',(66.9987790562313,-11.1664395775339,6.78144419148183));
#6727=CARTESIAN_POINT('Ctrl Pts',(66.9987790562313,-13.0463068270182,0.688029525576709));
#6728=CARTESIAN_POINT('Ctrl Pts',(66.9987790562313,-12.2630179722188,-4.50205714502921));
#6729=CARTESIAN_POINT('Ctrl Pts',(66.9987790562313,-8.67041284092607,-9.76871206154051));
#6730=CARTESIAN_POINT('Ctrl Pts',(66.9987790562313,-4.12713707506171,-12.3959020204541));
#6731=CARTESIAN_POINT('Ctrl Pts',(66.9987790562313,2.23105293326073,-12.8718884272354));
#6732=CARTESIAN_POINT('Ctrl Pts',(66.9987790562313,7.73425414613492,-10.7167983889895));
#6733=CARTESIAN_POINT('Ctrl Pts',(66.9987790562313,11.7564405197882,-5.65636604767626));
#6734=CARTESIAN_POINT('Ctrl Pts',(66.9987790562313,12.6177894202922,-1.88753252870586));
#6735=CARTESIAN_POINT('Ctrl Pts',(66.9987790562313,12.6177894202922,-4.44089209850063E-15));
#6736=CARTESIAN_POINT('Ctrl Pts',(66.9995926873144,12.6061681608754,8.28565575401122E-16));
#6737=CARTESIAN_POINT('Ctrl Pts',(66.9995926873144,12.6061681608754,1.88579407027011));
#6738=CARTESIAN_POINT('Ctrl Pts',(66.9995926873144,11.7457806031927,5.65649074488443));
#6739=CARTESIAN_POINT('Ctrl Pts',(66.9995926873144,8.12960304295226,10.191910765725));
#6740=CARTESIAN_POINT('Ctrl Pts',(66.9995926873143,2.8997823025916,12.7109430570306));
#6741=CARTESIAN_POINT('Ctrl Pts',(66.9995926873144,-2.25301447135012,12.7078965482737));
#6742=CARTESIAN_POINT('Ctrl Pts',(66.9995926873143,-7.58690347578576,10.6196890965696));
#6743=CARTESIAN_POINT('Ctrl Pts',(66.9995926873144,-11.1561550431592,6.77519833358192));
#6744=CARTESIAN_POINT('Ctrl Pts',(66.9995926873144,-13.0342908938368,0.687395835367529));
#6745=CARTESIAN_POINT('Ctrl Pts',(66.9995926873144,-12.2517234652816,-4.49791065210782));
#6746=CARTESIAN_POINT('Ctrl Pts',(66.9995926873144,-8.6624272014315,-9.75971486475775));
#6747=CARTESIAN_POINT('Ctrl Pts',(66.9995926873144,-4.12333589187291,-12.3844851243478));
#6748=CARTESIAN_POINT('Ctrl Pts',(66.9995926873143,2.22899808482832,-12.8600331372316));
#6749=CARTESIAN_POINT('Ctrl Pts',(66.9995926873144,7.7271307294426,-10.7069279839104));
#6750=CARTESIAN_POINT('Ctrl Pts',(66.9995926873144,11.745612581646,-5.65115641111024));
#6751=CARTESIAN_POINT('Ctrl Pts',(66.9995926873144,12.6061681608753,-1.88579407027012));
#6752=CARTESIAN_POINT('Ctrl Pts',(66.9995926873144,12.6061681608753,-4.43755947288309E-15));
#6753=CARTESIAN_POINT('Ctrl Pts',(67.,12.5945184588186,8.24916091886633E-16));
#6754=CARTESIAN_POINT('Ctrl Pts',(67.,12.5945184588186,1.88405135674166));
#6755=CARTESIAN_POINT('Ctrl Pts',(67.,11.7349260085885,5.65126342830562));
#6756=CARTESIAN_POINT('Ctrl Pts',(67.,8.12209025615349,10.1824921443827));
#6757=CARTESIAN_POINT('Ctrl Pts',(67.,2.89710253505555,12.6991965296307));
#6758=CARTESIAN_POINT('Ctrl Pts',(67.,-2.25093239955722,12.6961528361925));
#6759=CARTESIAN_POINT('Ctrl Pts',(67.,-7.57989221236772,10.6098751537225));
#6760=CARTESIAN_POINT('Ctrl Pts',(67.,-11.1458453375251,6.76893718890919));
#6761=CARTESIAN_POINT('Ctrl Pts',(67.,-13.0222455519134,0.686760594224371));
#6762=CARTESIAN_POINT('Ctrl Pts',(67.,-12.2404013151221,-4.49375401083788));
#6763=CARTESIAN_POINT('Ctrl Pts',(67.,-8.65442201741998,-9.75069564737116));
#6764=CARTESIAN_POINT('Ctrl Pts',(67.,-4.11952540525758,-12.3730402855533));
#6765=CARTESIAN_POINT('Ctrl Pts',(67.,2.22693820721373,-12.8481488316227));
#6766=CARTESIAN_POINT('Ctrl Pts',(67.,7.71998987822122,-10.6970334212052));
#6767=CARTESIAN_POINT('Ctrl Pts',(67.,11.7347581423126,-5.64593402412958));
#6768=CARTESIAN_POINT('Ctrl Pts',(67.,12.5945184588185,-1.88405135674167));
#6769=CARTESIAN_POINT('Ctrl Pts',(67.,12.5945184588185,-4.43377464066931E-15));
#6770=CARTESIAN_POINT('Ctrl Pts',(67.,12.5828687521281,8.21727726654077E-16));
#6771=CARTESIAN_POINT('Ctrl Pts',(67.,12.5828687521281,1.8823086424221));
#6772=CARTESIAN_POINT('Ctrl Pts',(67.,11.7240714096075,5.64603610965329));
#6773=CARTESIAN_POINT('Ctrl Pts',(67.,8.11457746630642,10.1730735192044));
#6774=CARTESIAN_POINT('Ctrl Pts',(67.,2.89442276640883,12.6874499975273));
#6775=CARTESIAN_POINT('Ctrl Pts',(67.,-2.24885032695964,12.6844091193373));
#6776=CARTESIAN_POINT('Ctrl Pts',(67.,-7.57288094607568,10.6000612069797));
#6777=CARTESIAN_POINT('Ctrl Pts',(67.,-11.1355356277156,6.76267604165808));
#6778=CARTESIAN_POINT('Ctrl Pts',(67.,-13.010200205145,0.686125352829048));
#6779=CARTESIAN_POINT('Ctrl Pts',(67.,-12.2290791603529,-4.48959736793348));
#6780=CARTESIAN_POINT('Ctrl Pts',(67.,-8.6464168302479,-9.7416764263013));
#6781=CARTESIAN_POINT('Ctrl Pts',(67.,-4.11571491706988,-12.3615954421279));
#6782=CARTESIAN_POINT('Ctrl Pts',(67.,2.22487832877622,-12.8362645212214));
#6783=CARTESIAN_POINT('Ctrl Pts',(67.,7.71284902408557,-10.6871388545133));
#6784=CARTESIAN_POINT('Ctrl Pts',(67.,11.723903698598,-5.64071163506987));
#6785=CARTESIAN_POINT('Ctrl Pts',(67.,12.5828687521281,-1.88230864242211));
#6786=CARTESIAN_POINT('Ctrl Pts',(67.,12.5828687521281,-4.42954684098673E-15));
#6787=CARTESIAN_POINT('',(66.9987790562313,12.6177894202923,-2.22044604925031E-15));
#6788=CARTESIAN_POINT('Origin',(66.5,12.5828687521281,1.38777878078145E-15));
#6789=CARTESIAN_POINT('Ctrl Pts',(66.9987790562313,12.6177894202923,8.32667268468867E-16));
#6790=CARTESIAN_POINT('Ctrl Pts',(66.9987790562313,12.6177894202923,1.88753252870585));
#6791=CARTESIAN_POINT('Ctrl Pts',(66.9987790562313,11.7566086962385,5.66170529903387));
#6792=CARTESIAN_POINT('Ctrl Pts',(66.9987790562313,8.13709748718362,10.2013063913397));
#6793=CARTESIAN_POINT('Ctrl Pts',(66.9987790562312,2.90245552737485,12.7226609053052));
#6794=CARTESIAN_POINT('Ctrl Pts',(66.9987790562313,-2.25509145984958,12.7196115879031));
#6795=CARTESIAN_POINT('Ctrl Pts',(66.9987790562313,-7.59389762103065,10.6294790787878));
#6796=CARTESIAN_POINT('Ctrl Pts',(66.9987790562313,-11.1664395775339,6.78144419148183));
#6797=CARTESIAN_POINT('Ctrl Pts',(66.9987790562313,-13.0463068270182,0.688029525576709));
#6798=CARTESIAN_POINT('Ctrl Pts',(66.9987790562313,-12.2630179722188,-4.50205714502921));
#6799=CARTESIAN_POINT('Ctrl Pts',(66.9987790562313,-8.67041284092607,-9.76871206154051));
#6800=CARTESIAN_POINT('Ctrl Pts',(66.9987790562313,-4.12713707506171,-12.3959020204541));
#6801=CARTESIAN_POINT('Ctrl Pts',(66.9987790562313,2.23105293326073,-12.8718884272354));
#6802=CARTESIAN_POINT('Ctrl Pts',(66.9987790562313,7.73425414613492,-10.7167983889895));
#6803=CARTESIAN_POINT('Ctrl Pts',(66.9987790562313,11.7564405197882,-5.65636604767626));
#6804=CARTESIAN_POINT('Ctrl Pts',(66.9987790562313,12.6177894202922,-1.88753252870586));
#6805=CARTESIAN_POINT('Ctrl Pts',(66.9987790562313,12.6177894202922,-4.44089209850063E-15));
#6806=CARTESIAN_POINT('Ctrl Pts',(67.,12.6,0.));
#6807=CARTESIAN_POINT('Ctrl Pts',(67.,12.6,12.6));
#6808=CARTESIAN_POINT('Ctrl Pts',(67.,0.,12.6));
#6809=CARTESIAN_POINT('Ctrl Pts',(67.,-12.6,12.6));
#6810=CARTESIAN_POINT('Ctrl Pts',(67.,-12.6,0.));
#6811=CARTESIAN_POINT('Ctrl Pts',(67.,-12.6,-12.6));
#6812=CARTESIAN_POINT('Ctrl Pts',(67.,0.,-12.6));
#6813=CARTESIAN_POINT('Ctrl Pts',(67.,12.6,-12.6));
#6814=CARTESIAN_POINT('Ctrl Pts',(67.,12.6,0.));
#6815=CARTESIAN_POINT('Ctrl Pts',(66.9932926583693,12.6997352662803,0.));
#6816=CARTESIAN_POINT('Ctrl Pts',(66.9932926583693,12.6997352662803,12.6997352662803));
#6817=CARTESIAN_POINT('Ctrl Pts',(66.9932926583693,0.,12.6997352662803));
#6818=CARTESIAN_POINT('Ctrl Pts',(66.9932926583693,-12.6997352662803,12.6997352662803));
#6819=CARTESIAN_POINT('Ctrl Pts',(66.9932926583693,-12.6997352662803,0.));
#6820=CARTESIAN_POINT('Ctrl Pts',(66.9932926583693,-12.6997352662803,-12.6997352662803));
#6821=CARTESIAN_POINT('Ctrl Pts',(66.9932926583693,0.,-12.6997352662803));
#6822=CARTESIAN_POINT('Ctrl Pts',(66.9932926583693,12.6997352662803,-12.6997352662803));
#6823=CARTESIAN_POINT('Ctrl Pts',(66.9932926583693,12.6997352662803,0.));
#6824=CARTESIAN_POINT('Ctrl Pts',(66.9758353862889,12.9017721172185,0.));
#6825=CARTESIAN_POINT('Ctrl Pts',(66.9758353862889,12.9017721172185,12.9017721172185));
#6826=CARTESIAN_POINT('Ctrl Pts',(66.9758353862889,0.,12.9017721172185));
#6827=CARTESIAN_POINT('Ctrl Pts',(66.9758353862889,-12.9017721172185,12.9017721172185));
#6828=CARTESIAN_POINT('Ctrl Pts',(66.9758353862889,-12.9017721172185,0.));
#6829=CARTESIAN_POINT('Ctrl Pts',(66.9758353862889,-12.9017721172185,-12.9017721172185));
#6830=CARTESIAN_POINT('Ctrl Pts',(66.9758353862889,0.,-12.9017721172185));
#6831=CARTESIAN_POINT('Ctrl Pts',(66.9758353862889,12.9017721172185,-12.9017721172185));
#6832=CARTESIAN_POINT('Ctrl Pts',(66.9758353862889,12.9017721172185,0.));
#6833=CARTESIAN_POINT('Ctrl Pts',(66.9375217173852,13.2125265684525,0.));
#6834=CARTESIAN_POINT('Ctrl Pts',(66.9375217173852,13.2125265684525,13.2125265684525));
#6835=CARTESIAN_POINT('Ctrl Pts',(66.9375217173852,0.,13.2125265684525));
#6836=CARTESIAN_POINT('Ctrl Pts',(66.9375217173852,-13.2125265684525,13.2125265684525));
#6837=CARTESIAN_POINT('Ctrl Pts',(66.9375217173852,-13.2125265684525,0.));
#6838=CARTESIAN_POINT('Ctrl Pts',(66.9375217173852,-13.2125265684525,-13.2125265684525));
#6839=CARTESIAN_POINT('Ctrl Pts',(66.9375217173852,0.,-13.2125265684525));
#6840=CARTESIAN_POINT('Ctrl Pts',(66.9375217173852,13.2125265684525,-13.2125265684525));
#6841=CARTESIAN_POINT('Ctrl Pts',(66.9375217173852,13.2125265684525,0.));
#6842=CARTESIAN_POINT('Ctrl Pts',(66.8621179770906,13.6423024645368,0.));
#6843=CARTESIAN_POINT('Ctrl Pts',(66.8621179770906,13.6423024645368,13.6423024645368));
#6844=CARTESIAN_POINT('Ctrl Pts',(66.8621179770906,0.,13.6423024645368));
#6845=CARTESIAN_POINT('Ctrl Pts',(66.8621179770906,-13.6423024645368,13.6423024645368));
#6846=CARTESIAN_POINT('Ctrl Pts',(66.8621179770906,-13.6423024645368,0.));
#6847=CARTESIAN_POINT('Ctrl Pts',(66.8621179770906,-13.6423024645368,-13.6423024645368));
#6848=CARTESIAN_POINT('Ctrl Pts',(66.8621179770906,0.,-13.6423024645368));
#6849=CARTESIAN_POINT('Ctrl Pts',(66.8621179770906,13.6423024645368,-13.6423024645368));
#6850=CARTESIAN_POINT('Ctrl Pts',(66.8621179770906,13.6423024645368,0.));
#6851=CARTESIAN_POINT('Ctrl Pts',(66.7270226914732,14.2049623954268,0.));
#6852=CARTESIAN_POINT('Ctrl Pts',(66.7270226914732,14.2049623954268,14.2049623954268));
#6853=CARTESIAN_POINT('Ctrl Pts',(66.7270226914732,0.,14.2049623954268));
#6854=CARTESIAN_POINT('Ctrl Pts',(66.7270226914732,-14.2049623954268,14.2049623954268));
#6855=CARTESIAN_POINT('Ctrl Pts',(66.7270226914732,-14.2049623954268,0.));
#6856=CARTESIAN_POINT('Ctrl Pts',(66.7270226914732,-14.2049623954268,-14.2049623954268));
#6857=CARTESIAN_POINT('Ctrl Pts',(66.7270226914732,0.,-14.2049623954268));
#6858=CARTESIAN_POINT('Ctrl Pts',(66.7270226914732,14.2049623954268,-14.2049623954268));
#6859=CARTESIAN_POINT('Ctrl Pts',(66.7270226914732,14.2049623954268,0.));
#6860=CARTESIAN_POINT('Ctrl Pts',(66.5508049999324,14.7917496047061,0.));
#6861=CARTESIAN_POINT('Ctrl Pts',(66.5508049999324,14.7917496047061,14.7917496047061));
#6862=CARTESIAN_POINT('Ctrl Pts',(66.5508049999324,0.,14.7917496047061));
#6863=CARTESIAN_POINT('Ctrl Pts',(66.5508049999324,-14.7917496047061,14.7917496047061));
#6864=CARTESIAN_POINT('Ctrl Pts',(66.5508049999324,-14.7917496047061,0.));
#6865=CARTESIAN_POINT('Ctrl Pts',(66.5508049999324,-14.7917496047061,-14.7917496047061));
#6866=CARTESIAN_POINT('Ctrl Pts',(66.5508049999324,0.,-14.7917496047061));
#6867=CARTESIAN_POINT('Ctrl Pts',(66.5508049999324,14.7917496047061,-14.7917496047061));
#6868=CARTESIAN_POINT('Ctrl Pts',(66.5508049999324,14.7917496047061,0.));
#6869=CARTESIAN_POINT('Ctrl Pts',(66.333400353284,15.3997739599779,0.));
#6870=CARTESIAN_POINT('Ctrl Pts',(66.333400353284,15.3997739599778,15.3997739599778));
#6871=CARTESIAN_POINT('Ctrl Pts',(66.333400353284,0.,15.3997739599779));
#6872=CARTESIAN_POINT('Ctrl Pts',(66.333400353284,-15.3997739599778,15.3997739599778));
#6873=CARTESIAN_POINT('Ctrl Pts',(66.333400353284,-15.3997739599779,0.));
#6874=CARTESIAN_POINT('Ctrl Pts',(66.333400353284,-15.3997739599778,-15.3997739599778));
#6875=CARTESIAN_POINT('Ctrl Pts',(66.333400353284,0.,-15.3997739599779));
#6876=CARTESIAN_POINT('Ctrl Pts',(66.333400353284,15.3997739599778,-15.3997739599778));
#6877=CARTESIAN_POINT('Ctrl Pts',(66.333400353284,15.3997739599779,0.));
#6878=CARTESIAN_POINT('Ctrl Pts',(66.0751703194864,16.0237534171383,0.));
#6879=CARTESIAN_POINT('Ctrl Pts',(66.0751703194864,16.0237534171383,16.0237534171383));
#6880=CARTESIAN_POINT('Ctrl Pts',(66.0751703194864,0.,16.0237534171383));
#6881=CARTESIAN_POINT('Ctrl Pts',(66.0751703194864,-16.0237534171383,16.0237534171383));
#6882=CARTESIAN_POINT('Ctrl Pts',(66.0751703194864,-16.0237534171383,0.));
#6883=CARTESIAN_POINT('Ctrl Pts',(66.0751703194864,-16.0237534171383,-16.0237534171383));
#6884=CARTESIAN_POINT('Ctrl Pts',(66.0751703194864,0.,-16.0237534171383));
#6885=CARTESIAN_POINT('Ctrl Pts',(66.0751703194864,16.0237534171383,-16.0237534171383));
#6886=CARTESIAN_POINT('Ctrl Pts',(66.0751703194864,16.0237534171383,0.));
#6887=CARTESIAN_POINT('Ctrl Pts',(65.7771152465929,16.6559365250315,0.));
#6888=CARTESIAN_POINT('Ctrl Pts',(65.7771152465929,16.6559365250315,16.6559365250315));
#6889=CARTESIAN_POINT('Ctrl Pts',(65.7771152465929,0.,16.6559365250315));
#6890=CARTESIAN_POINT('Ctrl Pts',(65.7771152465929,-16.6559365250315,16.6559365250315));
#6891=CARTESIAN_POINT('Ctrl Pts',(65.7771152465929,-16.6559365250315,0.));
#6892=CARTESIAN_POINT('Ctrl Pts',(65.7771152465929,-16.6559365250315,-16.6559365250315));
#6893=CARTESIAN_POINT('Ctrl Pts',(65.7771152465929,0.,-16.6559365250315));
#6894=CARTESIAN_POINT('Ctrl Pts',(65.7771152465929,16.6559365250315,-16.6559365250315));
#6895=CARTESIAN_POINT('Ctrl Pts',(65.7771152465929,16.6559365250315,0.));
#6896=CARTESIAN_POINT('Ctrl Pts',(65.4410849670182,17.2875976116165,0.));
#6897=CARTESIAN_POINT('Ctrl Pts',(65.4410849670182,17.2875976116165,17.2875976116165));
#6898=CARTESIAN_POINT('Ctrl Pts',(65.4410849670182,0.,17.2875976116165));
#6899=CARTESIAN_POINT('Ctrl Pts',(65.4410849670182,-17.2875976116165,17.2875976116165));
#6900=CARTESIAN_POINT('Ctrl Pts',(65.4410849670182,-17.2875976116165,0.));
#6901=CARTESIAN_POINT('Ctrl Pts',(65.4410849670182,-17.2875976116165,-17.2875976116165));
#6902=CARTESIAN_POINT('Ctrl Pts',(65.4410849670182,0.,-17.2875976116165));
#6903=CARTESIAN_POINT('Ctrl Pts',(65.4410849670182,17.2875976116165,-17.2875976116165));
#6904=CARTESIAN_POINT('Ctrl Pts',(65.4410849670182,17.2875976116165,0.));
#6905=CARTESIAN_POINT('Ctrl Pts',(65.0700058995025,17.9101691052111,0.));
#6906=CARTESIAN_POINT('Ctrl Pts',(65.0700058995025,17.9101691052111,17.9101691052111));
#6907=CARTESIAN_POINT('Ctrl Pts',(65.0700058995025,0.,17.9101691052111));
#6908=CARTESIAN_POINT('Ctrl Pts',(65.0700058995025,-17.9101691052111,17.9101691052111));
#6909=CARTESIAN_POINT('Ctrl Pts',(65.0700058995025,-17.9101691052111,0.));
#6910=CARTESIAN_POINT('Ctrl Pts',(65.0700058995025,-17.9101691052111,-17.9101691052111));
#6911=CARTESIAN_POINT('Ctrl Pts',(65.0700058995025,0.,-17.9101691052111));
#6912=CARTESIAN_POINT('Ctrl Pts',(65.0700058995025,17.9101691052111,-17.9101691052111));
#6913=CARTESIAN_POINT('Ctrl Pts',(65.0700058995025,17.9101691052111,0.));
#6914=CARTESIAN_POINT('Ctrl Pts',(64.6681449587856,18.5165543814796,0.));
#6915=CARTESIAN_POINT('Ctrl Pts',(64.6681449587856,18.5165543814796,18.5165543814796));
#6916=CARTESIAN_POINT('Ctrl Pts',(64.6681449587856,0.,18.5165543814796));
#6917=CARTESIAN_POINT('Ctrl Pts',(64.6681449587856,-18.5165543814796,18.5165543814796));
#6918=CARTESIAN_POINT('Ctrl Pts',(64.6681449587856,-18.5165543814796,0.));
#6919=CARTESIAN_POINT('Ctrl Pts',(64.6681449587856,-18.5165543814796,-18.5165543814796));
#6920=CARTESIAN_POINT('Ctrl Pts',(64.6681449587856,0.,-18.5165543814796));
#6921=CARTESIAN_POINT('Ctrl Pts',(64.6681449587856,18.5165543814796,-18.5165543814796));
#6922=CARTESIAN_POINT('Ctrl Pts',(64.6681449587856,18.5165543814796,0.));
#6923=CARTESIAN_POINT('Ctrl Pts',(64.241353075389,19.1022896867918,0.));
#6924=CARTESIAN_POINT('Ctrl Pts',(64.241353075389,19.1022896867918,19.1022896867918));
#6925=CARTESIAN_POINT('Ctrl Pts',(64.241353075389,0.,19.1022896867918));
#6926=CARTESIAN_POINT('Ctrl Pts',(64.241353075389,-19.1022896867918,19.1022896867918));
#6927=CARTESIAN_POINT('Ctrl Pts',(64.241353075389,-19.1022896867918,0.));
#6928=CARTESIAN_POINT('Ctrl Pts',(64.241353075389,-19.1022896867918,-19.1022896867918));
#6929=CARTESIAN_POINT('Ctrl Pts',(64.241353075389,0.,-19.1022896867918));
#6930=CARTESIAN_POINT('Ctrl Pts',(64.241353075389,19.1022896867918,-19.1022896867918));
#6931=CARTESIAN_POINT('Ctrl Pts',(64.241353075389,19.1022896867918,0.));
#6932=CARTESIAN_POINT('Ctrl Pts',(63.7974413872401,19.6670367803137,0.));
#6933=CARTESIAN_POINT('Ctrl Pts',(63.7974413872401,19.6670367803137,19.6670367803137));
#6934=CARTESIAN_POINT('Ctrl Pts',(63.7974413872401,0.,19.6670367803137));
#6935=CARTESIAN_POINT('Ctrl Pts',(63.7974413872401,-19.6670367803137,19.6670367803137));
#6936=CARTESIAN_POINT('Ctrl Pts',(63.7974413872401,-19.6670367803137,0.));
#6937=CARTESIAN_POINT('Ctrl Pts',(63.7974413872401,-19.6670367803137,-19.6670367803137));
#6938=CARTESIAN_POINT('Ctrl Pts',(63.7974413872401,0.,-19.6670367803137));
#6939=CARTESIAN_POINT('Ctrl Pts',(63.7974413872401,19.6670367803137,-19.6670367803137));
#6940=CARTESIAN_POINT('Ctrl Pts',(63.7974413872401,19.6670367803137,0.));
#6941=CARTESIAN_POINT('Ctrl Pts',(63.345612386475,20.2136468221279,0.));
#6942=CARTESIAN_POINT('Ctrl Pts',(63.345612386475,20.2136468221279,20.2136468221279));
#6943=CARTESIAN_POINT('Ctrl Pts',(63.345612386475,0.,20.2136468221279));
#6944=CARTESIAN_POINT('Ctrl Pts',(63.345612386475,-20.2136468221279,20.2136468221279));
#6945=CARTESIAN_POINT('Ctrl Pts',(63.345612386475,-20.2136468221279,0.));
#6946=CARTESIAN_POINT('Ctrl Pts',(63.345612386475,-20.2136468221279,-20.2136468221279));
#6947=CARTESIAN_POINT('Ctrl Pts',(63.345612386475,0.,-20.2136468221279));
#6948=CARTESIAN_POINT('Ctrl Pts',(63.345612386475,20.2136468221279,-20.2136468221279));
#6949=CARTESIAN_POINT('Ctrl Pts',(63.345612386475,20.2136468221279,0.));
#6950=CARTESIAN_POINT('Ctrl Pts',(62.8957596029255,20.7468804921309,0.));
#6951=CARTESIAN_POINT('Ctrl Pts',(62.8957596029255,20.7468804921309,20.7468804921309));
#6952=CARTESIAN_POINT('Ctrl Pts',(62.8957596029255,0.,20.7468804921309));
#6953=CARTESIAN_POINT('Ctrl Pts',(62.8957596029255,-20.7468804921309,20.7468804921309));
#6954=CARTESIAN_POINT('Ctrl Pts',(62.8957596029255,-20.7468804921309,0.));
#6955=CARTESIAN_POINT('Ctrl Pts',(62.8957596029255,-20.7468804921309,-20.7468804921309));
#6956=CARTESIAN_POINT('Ctrl Pts',(62.8957596029255,0.,-20.7468804921309));
#6957=CARTESIAN_POINT('Ctrl Pts',(62.8957596029255,20.7468804921309,-20.7468804921309));
#6958=CARTESIAN_POINT('Ctrl Pts',(62.8957596029255,20.7468804921309,0.));
#6959=CARTESIAN_POINT('Ctrl Pts',(62.4578085440914,21.2722425632023,0.));
#6960=CARTESIAN_POINT('Ctrl Pts',(62.4578085440914,21.2722425632023,21.2722425632023));
#6961=CARTESIAN_POINT('Ctrl Pts',(62.4578085440914,0.,21.2722425632023));
#6962=CARTESIAN_POINT('Ctrl Pts',(62.4578085440914,-21.2722425632023,21.2722425632023));
#6963=CARTESIAN_POINT('Ctrl Pts',(62.4578085440914,-21.2722425632023,0.));
#6964=CARTESIAN_POINT('Ctrl Pts',(62.4578085440914,-21.2722425632023,-21.2722425632023));
#6965=CARTESIAN_POINT('Ctrl Pts',(62.4578085440914,0.,-21.2722425632023));
#6966=CARTESIAN_POINT('Ctrl Pts',(62.4578085440914,21.2722425632023,-21.2722425632023));
#6967=CARTESIAN_POINT('Ctrl Pts',(62.4578085440914,21.2722425632023,0.));
#6968=CARTESIAN_POINT('Ctrl Pts',(62.0410846718656,21.7948710346798,0.));
#6969=CARTESIAN_POINT('Ctrl Pts',(62.0410846718656,21.7948710346798,21.7948710346798));
#6970=CARTESIAN_POINT('Ctrl Pts',(62.0410846718656,0.,21.7948710346798));
#6971=CARTESIAN_POINT('Ctrl Pts',(62.0410846718656,-21.7948710346798,21.7948710346798));
#6972=CARTESIAN_POINT('Ctrl Pts',(62.0410846718656,-21.7948710346798,0.));
#6973=CARTESIAN_POINT('Ctrl Pts',(62.0410846718656,-21.7948710346798,-21.7948710346798));
#6974=CARTESIAN_POINT('Ctrl Pts',(62.0410846718656,0.,-21.7948710346798));
#6975=CARTESIAN_POINT('Ctrl Pts',(62.0410846718656,21.7948710346798,-21.7948710346798));
#6976=CARTESIAN_POINT('Ctrl Pts',(62.0410846718656,21.7948710346798,0.));
#6977=CARTESIAN_POINT('Ctrl Pts',(61.6535606725113,22.3182034793593,0.));
#6978=CARTESIAN_POINT('Ctrl Pts',(61.6535606725113,22.3182034793593,22.3182034793593));
#6979=CARTESIAN_POINT('Ctrl Pts',(61.6535606725113,0.,22.3182034793593));
#6980=CARTESIAN_POINT('Ctrl Pts',(61.6535606725113,-22.3182034793593,22.3182034793593));
#6981=CARTESIAN_POINT('Ctrl Pts',(61.6535606725113,-22.3182034793593,0.));
#6982=CARTESIAN_POINT('Ctrl Pts',(61.6535606725113,-22.3182034793593,-22.3182034793593));
#6983=CARTESIAN_POINT('Ctrl Pts',(61.6535606725113,0.,-22.3182034793593));
#6984=CARTESIAN_POINT('Ctrl Pts',(61.6535606725113,22.3182034793593,-22.3182034793593));
#6985=CARTESIAN_POINT('Ctrl Pts',(61.6535606725113,22.3182034793593,0.));
#6986=CARTESIAN_POINT('Ctrl Pts',(61.3014818178065,22.8434269247565,0.));
#6987=CARTESIAN_POINT('Ctrl Pts',(61.3014818178065,22.8434269247565,22.8434269247565));
#6988=CARTESIAN_POINT('Ctrl Pts',(61.3014818178065,0.,22.8434269247565));
#6989=CARTESIAN_POINT('Ctrl Pts',(61.3014818178065,-22.8434269247565,22.8434269247565));
#6990=CARTESIAN_POINT('Ctrl Pts',(61.3014818178065,-22.8434269247565,0.));
#6991=CARTESIAN_POINT('Ctrl Pts',(61.3014818178065,-22.8434269247565,-22.8434269247565));
#6992=CARTESIAN_POINT('Ctrl Pts',(61.3014818178065,0.,-22.8434269247565));
#6993=CARTESIAN_POINT('Ctrl Pts',(61.3014818178065,22.8434269247565,-22.8434269247565));
#6994=CARTESIAN_POINT('Ctrl Pts',(61.3014818178065,22.8434269247565,0.));
#6995=CARTESIAN_POINT('Ctrl Pts',(60.9896656117218,23.370292675902,0.));
#6996=CARTESIAN_POINT('Ctrl Pts',(60.9896656117218,23.370292675902,23.370292675902));
#6997=CARTESIAN_POINT('Ctrl Pts',(60.9896656117218,0.,23.370292675902));
#6998=CARTESIAN_POINT('Ctrl Pts',(60.9896656117218,-23.370292675902,23.370292675902));
#6999=CARTESIAN_POINT('Ctrl Pts',(60.9896656117218,-23.370292675902,0.));
#7000=CARTESIAN_POINT('Ctrl Pts',(60.9896656117218,-23.370292675902,-23.370292675902));
#7001=CARTESIAN_POINT('Ctrl Pts',(60.9896656117218,0.,-23.370292675902));
#7002=CARTESIAN_POINT('Ctrl Pts',(60.9896656117218,23.370292675902,-23.370292675902));
#7003=CARTESIAN_POINT('Ctrl Pts',(60.9896656117218,23.370292675902,0.));
#7004=CARTESIAN_POINT('Ctrl Pts',(60.7216146343454,23.8976229480199,0.));
#7005=CARTESIAN_POINT('Ctrl Pts',(60.7216146343454,23.8976229480199,23.8976229480199));
#7006=CARTESIAN_POINT('Ctrl Pts',(60.7216146343454,0.,23.8976229480199));
#7007=CARTESIAN_POINT('Ctrl Pts',(60.7216146343454,-23.8976229480199,23.8976229480199));
#7008=CARTESIAN_POINT('Ctrl Pts',(60.7216146343454,-23.8976229480199,0.));
#7009=CARTESIAN_POINT('Ctrl Pts',(60.7216146343454,-23.8976229480199,-23.8976229480199));
#7010=CARTESIAN_POINT('Ctrl Pts',(60.7216146343454,0.,-23.8976229480199));
#7011=CARTESIAN_POINT('Ctrl Pts',(60.7216146343454,23.8976229480199,-23.8976229480199));
#7012=CARTESIAN_POINT('Ctrl Pts',(60.7216146343454,23.8976229480199,0.));
#7013=CARTESIAN_POINT('Ctrl Pts',(60.4996857760211,24.4238918300188,0.));
#7014=CARTESIAN_POINT('Ctrl Pts',(60.4996857760211,24.4238918300188,24.4238918300188));
#7015=CARTESIAN_POINT('Ctrl Pts',(60.4996857760211,0.,24.4238918300188));
#7016=CARTESIAN_POINT('Ctrl Pts',(60.4996857760211,-24.4238918300188,24.4238918300188));
#7017=CARTESIAN_POINT('Ctrl Pts',(60.4996857760211,-24.4238918300188,0.));
#7018=CARTESIAN_POINT('Ctrl Pts',(60.4996857760211,-24.4238918300188,-24.4238918300188));
#7019=CARTESIAN_POINT('Ctrl Pts',(60.4996857760211,0.,-24.4238918300188));
#7020=CARTESIAN_POINT('Ctrl Pts',(60.4996857760211,24.4238918300188,-24.4238918300188));
#7021=CARTESIAN_POINT('Ctrl Pts',(60.4996857760211,24.4238918300188,0.));
#7022=CARTESIAN_POINT('Ctrl Pts',(60.3251702155445,24.947858058,0.));
#7023=CARTESIAN_POINT('Ctrl Pts',(60.3251702155445,24.947858058,24.947858058));
#7024=CARTESIAN_POINT('Ctrl Pts',(60.3251702155445,0.,24.947858058));
#7025=CARTESIAN_POINT('Ctrl Pts',(60.3251702155445,-24.947858058,24.947858058));
#7026=CARTESIAN_POINT('Ctrl Pts',(60.3251702155445,-24.947858058,0.));
#7027=CARTESIAN_POINT('Ctrl Pts',(60.3251702155445,-24.947858058,-24.947858058));
#7028=CARTESIAN_POINT('Ctrl Pts',(60.3251702155445,0.,-24.947858058));
#7029=CARTESIAN_POINT('Ctrl Pts',(60.3251702155445,24.947858058,-24.947858058));
#7030=CARTESIAN_POINT('Ctrl Pts',(60.3251702155445,24.947858058,0.));
#7031=CARTESIAN_POINT('Ctrl Pts',(60.1984961951092,25.4688514249257,0.));
#7032=CARTESIAN_POINT('Ctrl Pts',(60.1984961951092,25.4688514249257,25.4688514249257));
#7033=CARTESIAN_POINT('Ctrl Pts',(60.1984961951092,0.,25.4688514249257));
#7034=CARTESIAN_POINT('Ctrl Pts',(60.1984961951092,-25.4688514249257,25.4688514249257));
#7035=CARTESIAN_POINT('Ctrl Pts',(60.1984961951092,-25.4688514249257,0.));
#7036=CARTESIAN_POINT('Ctrl Pts',(60.1984961951092,-25.4688514249257,-25.4688514249257));
#7037=CARTESIAN_POINT('Ctrl Pts',(60.1984961951092,0.,-25.4688514249257));
#7038=CARTESIAN_POINT('Ctrl Pts',(60.1984961951092,25.4688514249257,-25.4688514249257));
#7039=CARTESIAN_POINT('Ctrl Pts',(60.1984961951092,25.4688514249257,0.));
#7040=CARTESIAN_POINT('Ctrl Pts',(60.1353708288129,25.8830038831508,0.));
#7041=CARTESIAN_POINT('Ctrl Pts',(60.1353708288129,25.8830038831508,25.8830038831508));
#7042=CARTESIAN_POINT('Ctrl Pts',(60.1353708288129,0.,25.8830038831508));
#7043=CARTESIAN_POINT('Ctrl Pts',(60.1353708288129,-25.8830038831508,25.8830038831508));
#7044=CARTESIAN_POINT('Ctrl Pts',(60.1353708288129,-25.8830038831508,0.));
#7045=CARTESIAN_POINT('Ctrl Pts',(60.1353708288129,-25.8830038831508,-25.8830038831508));
#7046=CARTESIAN_POINT('Ctrl Pts',(60.1353708288129,0.,-25.8830038831508));
#7047=CARTESIAN_POINT('Ctrl Pts',(60.1353708288129,25.8830038831508,-25.8830038831508));
#7048=CARTESIAN_POINT('Ctrl Pts',(60.1353708288129,25.8830038831508,0.));
#7049=CARTESIAN_POINT('Ctrl Pts',(60.1093965237418,26.1920935983768,0.));
#7050=CARTESIAN_POINT('Ctrl Pts',(60.1093965237418,26.1920935983768,26.1920935983768));
#7051=CARTESIAN_POINT('Ctrl Pts',(60.1093965237418,0.,26.1920935983768));
#7052=CARTESIAN_POINT('Ctrl Pts',(60.1093965237418,-26.1920935983768,26.1920935983768));
#7053=CARTESIAN_POINT('Ctrl Pts',(60.1093965237418,-26.1920935983768,0.));
#7054=CARTESIAN_POINT('Ctrl Pts',(60.1093965237418,-26.1920935983768,-26.1920935983768));
#7055=CARTESIAN_POINT('Ctrl Pts',(60.1093965237418,0.,-26.1920935983768));
#7056=CARTESIAN_POINT('Ctrl Pts',(60.1093965237418,26.1920935983768,-26.1920935983768));
#7057=CARTESIAN_POINT('Ctrl Pts',(60.1093965237418,26.1920935983768,0.));
#7058=CARTESIAN_POINT('Ctrl Pts',(60.1015533409406,26.3974772180319,0.));
#7059=CARTESIAN_POINT('Ctrl Pts',(60.1015533409406,26.3974772180319,26.3974772180319));
#7060=CARTESIAN_POINT('Ctrl Pts',(60.1015533409406,0.,26.3974772180319));
#7061=CARTESIAN_POINT('Ctrl Pts',(60.1015533409406,-26.3974772180319,26.3974772180319));
#7062=CARTESIAN_POINT('Ctrl Pts',(60.1015533409406,-26.3974772180319,0.));
#7063=CARTESIAN_POINT('Ctrl Pts',(60.1015533409406,-26.3974772180319,-26.3974772180319));
#7064=CARTESIAN_POINT('Ctrl Pts',(60.1015533409406,0.,-26.3974772180319));
#7065=CARTESIAN_POINT('Ctrl Pts',(60.1015533409406,26.3974772180319,-26.3974772180319));
#7066=CARTESIAN_POINT('Ctrl Pts',(60.1015533409406,26.3974772180319,0.));
#7067=CARTESIAN_POINT('Ctrl Pts',(60.1,26.5,0.));
#7068=CARTESIAN_POINT('Ctrl Pts',(60.1,26.5,26.5));
#7069=CARTESIAN_POINT('Ctrl Pts',(60.1,0.,26.5));
#7070=CARTESIAN_POINT('Ctrl Pts',(60.1,-26.5,26.5));
#7071=CARTESIAN_POINT('Ctrl Pts',(60.1,-26.5,0.));
#7072=CARTESIAN_POINT('Ctrl Pts',(60.1,-26.5,-26.5));
#7073=CARTESIAN_POINT('Ctrl Pts',(60.1,0.,-26.5));
#7074=CARTESIAN_POINT('Ctrl Pts',(60.1,26.5,-26.5));
#7075=CARTESIAN_POINT('Ctrl Pts',(60.1,26.5,0.));
#7076=CARTESIAN_POINT('',(60.1000630537694,26.4959364690653,9.43689570931383E-15));
#7077=CARTESIAN_POINT('Ctrl Pts',(66.9987790562313,12.6177894202923,0.));
#7078=CARTESIAN_POINT('Ctrl Pts',(66.9920328774672,12.714146473408,0.));
#7079=CARTESIAN_POINT('Ctrl Pts',(66.9744621413525,12.9128524924851,0.));
#7080=CARTESIAN_POINT('Ctrl Pts',(66.9361754064266,13.2201869184335,0.));
#7081=CARTESIAN_POINT('Ctrl Pts',(66.8611550018322,13.6463131714231,0.));
#7082=CARTESIAN_POINT('Ctrl Pts',(66.7270226914732,14.2049623954268,0.));
#7083=CARTESIAN_POINT('Ctrl Pts',(66.5508049999324,14.7917496047061,0.));
#7084=CARTESIAN_POINT('Ctrl Pts',(66.333400353284,15.3997739599779,0.));
#7085=CARTESIAN_POINT('Ctrl Pts',(66.0751703194864,16.0237534171383,0.));
#7086=CARTESIAN_POINT('Ctrl Pts',(65.7771152465929,16.6559365250315,0.));
#7087=CARTESIAN_POINT('Ctrl Pts',(65.4410849670182,17.2875976116165,0.));
#7088=CARTESIAN_POINT('Ctrl Pts',(65.0700058995025,17.9101691052111,0.));
#7089=CARTESIAN_POINT('Ctrl Pts',(64.6681449587856,18.5165543814796,0.));
#7090=CARTESIAN_POINT('Ctrl Pts',(64.241353075389,19.1022896867918,0.));
#7091=CARTESIAN_POINT('Ctrl Pts',(63.7974413872401,19.6670367803137,0.));
#7092=CARTESIAN_POINT('Ctrl Pts',(63.345612386475,20.2136468221279,0.));
#7093=CARTESIAN_POINT('Ctrl Pts',(62.8957596029255,20.7468804921309,0.));
#7094=CARTESIAN_POINT('Ctrl Pts',(62.4578085440914,21.2722425632023,0.));
#7095=CARTESIAN_POINT('Ctrl Pts',(62.0410846718656,21.7948710346798,0.));
#7096=CARTESIAN_POINT('Ctrl Pts',(61.6535606725113,22.3182034793593,0.));
#7097=CARTESIAN_POINT('Ctrl Pts',(61.3014818178065,22.8434269247565,0.));
#7098=CARTESIAN_POINT('Ctrl Pts',(60.9896656117218,23.370292675902,0.));
#7099=CARTESIAN_POINT('Ctrl Pts',(60.7216146343454,23.8976229480199,0.));
#7100=CARTESIAN_POINT('Ctrl Pts',(60.4996857760211,24.4238918300188,0.));
#7101=CARTESIAN_POINT('Ctrl Pts',(60.3251702155445,24.947858058,0.));
#7102=CARTESIAN_POINT('Ctrl Pts',(60.1986970208453,25.4680254554329,0.));
#7103=CARTESIAN_POINT('Ctrl Pts',(60.1356211722196,25.8813624061185,0.));
#7104=CARTESIAN_POINT('Ctrl Pts',(60.1096028663132,26.1896434519942,0.));
#7105=CARTESIAN_POINT('Ctrl Pts',(60.101678577611,26.3942210551826,0.));
#7106=CARTESIAN_POINT('Ctrl Pts',(60.1000630537672,26.4959364692063,0.));
#7107=CARTESIAN_POINT('Ctrl Pts',(60.1000630537694,26.4959364690656,1.88737914186277E-14));
#7108=CARTESIAN_POINT('Ctrl Pts',(60.1000630537694,26.4959364690656,-3.9636056917746));
#7109=CARTESIAN_POINT('Ctrl Pts',(60.1000630537694,24.685961262727,-11.8807347957342));
#7110=CARTESIAN_POINT('Ctrl Pts',(60.1000630537695,16.2443369841089,-22.4988484266417));
#7111=CARTESIAN_POINT('Ctrl Pts',(60.1000630537694,4.68027293296291,-27.0375433673444));
#7112=CARTESIAN_POINT('Ctrl Pts',(60.1000630537694,-5.98560140555878,-26.2137571448923));
#7113=CARTESIAN_POINT('Ctrl Pts',(60.1000630537694,-13.4488703508335,-23.2938884734323));
#7114=CARTESIAN_POINT('Ctrl Pts',(60.1000630537694,-19.7110570984953,-18.2910903026092));
#7115=CARTESIAN_POINT('Ctrl Pts',(60.1000630537694,-25.752819385365,-9.46432907623452));
#7116=CARTESIAN_POINT('Ctrl Pts',(60.1000630537694,-27.4017087341173,1.45271682099757));
#7117=CARTESIAN_POINT('Ctrl Pts',(60.1000630537694,-24.2241191010755,11.6698194289465));
#7118=CARTESIAN_POINT('Ctrl Pts',(60.1000630537694,-19.717439049817,18.2934039326558));
#7119=CARTESIAN_POINT('Ctrl Pts',(60.1000630537694,-13.4457047614966,23.2905009850213));
#7120=CARTESIAN_POINT('Ctrl Pts',(60.1000630537694,-4.74183848087839,26.7134634764109));
#7121=CARTESIAN_POINT('Ctrl Pts',(60.1000630537694,6.09759643163882,26.714979249407));
#7122=CARTESIAN_POINT('Ctrl Pts',(60.1000630537694,17.0850948456638,21.4229364239694));
#7123=CARTESIAN_POINT('Ctrl Pts',(60.1000630537694,24.6887294488487,11.8885228778762));
#7124=CARTESIAN_POINT('Ctrl Pts',(60.1000630537694,26.4959364690658,3.9636056917746));
#7125=CARTESIAN_POINT('Ctrl Pts',(60.1000630537694,26.4959364690658,-1.72084568816899E-14));
#7126=CARTESIAN_POINT('Ctrl Pts',(60.1000630537694,26.4959364690658,-1.72084568816899E-14));
#7127=CARTESIAN_POINT('Ctrl Pts',(60.1000630537694,26.4959364690658,3.9636056917746));
#7128=CARTESIAN_POINT('Ctrl Pts',(60.1000630537694,24.6887294488487,11.8885228778762));
#7129=CARTESIAN_POINT('Ctrl Pts',(60.1000630537694,17.0850948456638,21.4229364239694));
#7130=CARTESIAN_POINT('Ctrl Pts',(60.1000630537694,6.09759643163882,26.714979249407));
#7131=CARTESIAN_POINT('Ctrl Pts',(60.1000630537694,-4.74183848087839,26.7134634764109));
#7132=CARTESIAN_POINT('Ctrl Pts',(60.1000630537694,-13.4457047614966,23.2905009850213));
#7133=CARTESIAN_POINT('Ctrl Pts',(60.1000630537694,-19.717439049817,18.2934039326558));
#7134=CARTESIAN_POINT('Ctrl Pts',(60.1000630537694,-24.2241191010755,11.6698194289465));
#7135=CARTESIAN_POINT('Ctrl Pts',(60.1000630537694,-27.4017087341173,1.45271682099757));
#7136=CARTESIAN_POINT('Ctrl Pts',(60.1000630537694,-25.752819385365,-9.46432907623452));
#7137=CARTESIAN_POINT('Ctrl Pts',(60.1000630537694,-19.7110570984953,-18.2910903026092));
#7138=CARTESIAN_POINT('Ctrl Pts',(60.1000630537694,-13.4488703508335,-23.2938884734323));
#7139=CARTESIAN_POINT('Ctrl Pts',(60.1000630537694,-5.98560140555878,-26.2137571448923));
#7140=CARTESIAN_POINT('Ctrl Pts',(60.1000630537694,4.68027293296291,-27.0375433673444));
#7141=CARTESIAN_POINT('Ctrl Pts',(60.1000630537695,16.2443369841089,-22.4988484266417));
#7142=CARTESIAN_POINT('Ctrl Pts',(60.1000630537694,24.685961262727,-11.8807347957342));
#7143=CARTESIAN_POINT('Ctrl Pts',(60.1000630537694,26.4959364690656,-3.9636056917746));
#7144=CARTESIAN_POINT('Ctrl Pts',(60.1000630537694,26.4959364690656,1.88737914186277E-14));
#7145=CARTESIAN_POINT('Ctrl Pts',(60.1000210188067,26.4985830432097,-1.72080134116452E-14));
#7146=CARTESIAN_POINT('Ctrl Pts',(60.1000210188067,26.4985830432097,3.96400160064724));
#7147=CARTESIAN_POINT('Ctrl Pts',(60.1000210188067,24.6911955082417,11.8897103753363));
#7148=CARTESIAN_POINT('Ctrl Pts',(60.1000210188067,17.0868014081141,21.4250762762329));
#7149=CARTESIAN_POINT('Ctrl Pts',(60.1000210188067,6.09820549639387,26.7176477028667));
#7150=CARTESIAN_POINT('Ctrl Pts',(60.1000210188066,-4.74231212434193,26.716131778466));
#7151=CARTESIAN_POINT('Ctrl Pts',(60.1000210188067,-13.4470477996871,23.2928273809114));
#7152=CARTESIAN_POINT('Ctrl Pts',(60.1000210188066,-19.7194085467032,18.2952311883147));
#7153=CARTESIAN_POINT('Ctrl Pts',(60.1000210188067,-24.2265387523811,11.6709850809853));
#7154=CARTESIAN_POINT('Ctrl Pts',(60.1000210188066,-27.404445782265,1.45286192712664));
#7155=CARTESIAN_POINT('Ctrl Pts',(60.1000210188067,-25.7553917324869,-9.46527443057792));
#7156=CARTESIAN_POINT('Ctrl Pts',(60.1000210188066,-19.7130259579137,-18.2929173271688));
#7157=CARTESIAN_POINT('Ctrl Pts',(60.1000210188067,-13.4502137052222,-23.2962152076852));
#7158=CARTESIAN_POINT('Ctrl Pts',(60.1000210188067,-5.98619928357432,-26.2163755332612));
#7159=CARTESIAN_POINT('Ctrl Pts',(60.1000210188067,4.6807404268877,-27.0402440404561));
#7160=CARTESIAN_POINT('Ctrl Pts',(60.1000210188067,16.2459595665867,-22.5010957474934));
#7161=CARTESIAN_POINT('Ctrl Pts',(60.1000210188067,24.6884270456168,-11.8819215152736));
#7162=CARTESIAN_POINT('Ctrl Pts',(60.1000210188067,26.4985830432095,-3.96400160064724));
#7163=CARTESIAN_POINT('Ctrl Pts',(60.1000210188067,26.4985830432095,1.88736805511165E-14));
#7164=CARTESIAN_POINT('Ctrl Pts',(60.1,26.5012299511459,-1.72076166127272E-14));
#7165=CARTESIAN_POINT('Ctrl Pts',(60.1,26.5012299511459,3.96439755945304));
#7166=CARTESIAN_POINT('Ctrl Pts',(60.1,24.6936618786601,11.8908980225664));
#7167=CARTESIAN_POINT('Ctrl Pts',(60.1,17.0885081858003,21.4272163983797));
#7168=CARTESIAN_POINT('Ctrl Pts',(60.1,6.09881463796566,26.720316492878));
#7169=CARTESIAN_POINT('Ctrl Pts',(60.1,-4.74278582754248,26.7188004170537));
#7170=CARTESIAN_POINT('Ctrl Pts',(60.1,-13.4483910072647,23.2951540702122));
#7171=CARTESIAN_POINT('Ctrl Pts',(60.1,-19.7213782919872,18.2970586744316));
#7172=CARTESIAN_POINT('Ctrl Pts',(60.1,-24.2289587088591,11.6721508800389));
#7173=CARTESIAN_POINT('Ctrl Pts',(60.1,-27.4071831756158,1.45300705155683));
#7174=CARTESIAN_POINT('Ctrl Pts',(60.1,-25.7579644040394,-9.46621990415165));
#7175=CARTESIAN_POINT('Ctrl Pts',(60.1,-19.7149950656494,-18.2947445821571));
#7176=CARTESIAN_POINT('Ctrl Pts',(60.1,-13.4515572290378,-23.2985422353914));
#7177=CARTESIAN_POINT('Ctrl Pts',(60.1,-5.98679723699566,-26.2189942518676));
#7178=CARTESIAN_POINT('Ctrl Pts',(60.1,4.68120797977395,-27.0429450541832));
#7179=CARTESIAN_POINT('Ctrl Pts',(60.1,16.2475823537085,-22.5033433517827));
#7180=CARTESIAN_POINT('Ctrl Pts',(60.1,24.6908931394971,-11.8831083844848));
#7181=CARTESIAN_POINT('Ctrl Pts',(60.1,26.5012299511458,-3.96439755945305));
#7182=CARTESIAN_POINT('Ctrl Pts',(60.1,26.5012299511458,1.88735230124792E-14));
#7183=CARTESIAN_POINT('Ctrl Pts',(60.1,26.503876859085,-1.72072665349743E-14));
#7184=CARTESIAN_POINT('Ctrl Pts',(60.1,26.503876859085,3.9647935182593));
#7185=CARTESIAN_POINT('Ctrl Pts',(60.1,24.6961282490811,11.8920856697977));
#7186=CARTESIAN_POINT('Ctrl Pts',(60.1,17.0902149634882,21.4293565205288));
#7187=CARTESIAN_POINT('Ctrl Pts',(60.1,6.09942377953813,26.7229852828923));
#7188=CARTESIAN_POINT('Ctrl Pts',(60.1,-4.74325953074353,26.7214690556444));
#7189=CARTESIAN_POINT('Ctrl Pts',(60.1,-13.4497342148437,23.2974807595154));
#7190=CARTESIAN_POINT('Ctrl Pts',(60.1,-19.7233480372732,18.2988861605503));
#7191=CARTESIAN_POINT('Ctrl Pts',(60.1,-24.2313786653396,11.6733166790938));
#7192=CARTESIAN_POINT('Ctrl Pts',(60.1,-27.4099205689696,1.45315217598718));
#7193=CARTESIAN_POINT('Ctrl Pts',(60.1,-25.7605370755947,-9.46716537772638));
#7194=CARTESIAN_POINT('Ctrl Pts',(60.1,-19.7169641733872,-18.2965718371474));
#7195=CARTESIAN_POINT('Ctrl Pts',(60.1,-13.4529007528549,-23.3008692631002));
#7196=CARTESIAN_POINT('Ctrl Pts',(60.1,-5.98739519041764,-26.2216129704768));
#7197=CARTESIAN_POINT('Ctrl Pts',(60.1,4.68167553266069,-27.0456460679132));
#7198=CARTESIAN_POINT('Ctrl Pts',(60.1,16.249205140832,-22.5055909560744));
#7199=CARTESIAN_POINT('Ctrl Pts',(60.1,24.6933592333801,-11.8842952536973));
#7200=CARTESIAN_POINT('Ctrl Pts',(60.1,26.5038768590848,-3.9647935182593));
#7201=CARTESIAN_POINT('Ctrl Pts',(60.1,26.5038768590848,1.88733188225822E-14));
#7202=CARTESIAN_POINT('',(60.1,26.503876859085,-1.83186799063151E-14));
#7203=CARTESIAN_POINT('Origin',(60.6,26.503876859085,-1.83186799063151E-14));
#7204=CARTESIAN_POINT('Ctrl Pts',(60.1,26.503876859085,-1.72072665349743E-14));
#7205=CARTESIAN_POINT('Ctrl Pts',(60.1,26.503876859085,3.9647935182593));
#7206=CARTESIAN_POINT('Ctrl Pts',(60.1,24.6961282490811,11.8920856697977));
#7207=CARTESIAN_POINT('Ctrl Pts',(60.1,17.0902149634882,21.4293565205288));
#7208=CARTESIAN_POINT('Ctrl Pts',(60.1,6.09942377953813,26.7229852828923));
#7209=CARTESIAN_POINT('Ctrl Pts',(60.1,-4.74325953074353,26.7214690556444));
#7210=CARTESIAN_POINT('Ctrl Pts',(60.1,-13.4497342148437,23.2974807595154));
#7211=CARTESIAN_POINT('Ctrl Pts',(60.1,-19.7233480372732,18.2988861605503));
#7212=CARTESIAN_POINT('Ctrl Pts',(60.1,-24.2313786653396,11.6733166790938));
#7213=CARTESIAN_POINT('Ctrl Pts',(60.1,-27.4099205689696,1.45315217598718));
#7214=CARTESIAN_POINT('Ctrl Pts',(60.1,-25.7605370755947,-9.46716537772638));
#7215=CARTESIAN_POINT('Ctrl Pts',(60.1,-19.7169641733872,-18.2965718371474));
#7216=CARTESIAN_POINT('Ctrl Pts',(60.1,-13.4529007528549,-23.3008692631002));
#7217=CARTESIAN_POINT('Ctrl Pts',(60.1,-5.98739519041764,-26.2216129704768));
#7218=CARTESIAN_POINT('Ctrl Pts',(60.1,4.68167553266069,-27.0456460679132));
#7219=CARTESIAN_POINT('Ctrl Pts',(60.1,16.249205140832,-22.5055909560744));
#7220=CARTESIAN_POINT('Ctrl Pts',(60.1,24.6933592333801,-11.8842952536973));
#7221=CARTESIAN_POINT('Ctrl Pts',(60.1,26.5038768590848,-3.9647935182593));
#7222=CARTESIAN_POINT('Ctrl Pts',(60.1,26.5038768590848,1.88733188225822E-14));
#7223=CARTESIAN_POINT('Origin',(60.1,26.5,0.));
#7224=CARTESIAN_POINT('',(60.1,57.4230311248647,-2.97413793103448));
#7225=CARTESIAN_POINT('',(60.1,57.4230311248647,2.97413793103448));
#7226=CARTESIAN_POINT('Origin',(60.1,0.,0.));
#7227=CARTESIAN_POINT('Origin',(60.1,0.,0.));
#7228=CARTESIAN_POINT('Ctrl Pts',(58.1000072797208,25.4986314827289,2.38697950294409E-14));
#7229=CARTESIAN_POINT('Ctrl Pts',(58.1000072797208,25.4986314827289,3.81441588205112));
#7230=CARTESIAN_POINT('Ctrl Pts',(58.1000072797208,23.7594464132255,11.4410395120049));
#7231=CARTESIAN_POINT('Ctrl Pts',(58.1000072797208,16.4420132235113,20.6165782938419));
#7232=CARTESIAN_POINT('Ctrl Pts',(58.1000072797208,5.8680831928706,25.709427795297));
#7233=CARTESIAN_POINT('Ctrl Pts',(58.1000072797208,-4.56335585676364,25.7079717649665));
#7234=CARTESIAN_POINT('Ctrl Pts',(58.1000072797208,-12.9396099811428,22.4138494830494));
#7235=CARTESIAN_POINT('Ctrl Pts',(58.1000072797208,-18.9752754976121,17.6048416816306));
#7236=CARTESIAN_POINT('Ctrl Pts',(58.1000072797208,-23.3123262403551,11.2305682370571));
#7237=CARTESIAN_POINT('Ctrl Pts',(58.1000072797208,-26.3703094632176,1.3980365463646));
#7238=CARTESIAN_POINT('Ctrl Pts',(58.1000072797208,-24.7834831225059,-9.10809204222051));
#7239=CARTESIAN_POINT('Ctrl Pts',(58.1000072797208,-18.9691368355184,-17.602615750836));
#7240=CARTESIAN_POINT('Ctrl Pts',(58.1000072797208,-12.9426554227937,-22.4171076785279));
#7241=CARTESIAN_POINT('Ctrl Pts',(58.1000072797208,-5.76030348627288,-25.2270747172432));
#7242=CARTESIAN_POINT('Ctrl Pts',(58.1000072797208,4.50410772030096,-26.0198514690206));
#7243=CARTESIAN_POINT('Ctrl Pts',(58.1000072797208,15.6329016549998,-21.6519940090828));
#7244=CARTESIAN_POINT('Ctrl Pts',(58.1000072797208,23.7567819506992,-11.4335435336754));
#7245=CARTESIAN_POINT('Ctrl Pts',(58.1000072797208,25.4986314827281,-3.81441588205099));
#7246=CARTESIAN_POINT('Ctrl Pts',(58.1000072797208,25.4986314827281,7.66053886991358E-14));
#7247=CARTESIAN_POINT('Ctrl Pts',(58.1000024265854,25.4995308359835,2.3870421523717E-14));
#7248=CARTESIAN_POINT('Ctrl Pts',(58.1000024265854,25.4995308359835,3.81455041897088));
#7249=CARTESIAN_POINT('Ctrl Pts',(58.1000024265854,23.7602844242958,11.4414430448819));
#7250=CARTESIAN_POINT('Ctrl Pts',(58.1000024265854,16.4425931439715,20.6173054539171));
#7251=CARTESIAN_POINT('Ctrl Pts',(58.1000024265854,5.86829016396711,25.7103345834742));
#7252=CARTESIAN_POINT('Ctrl Pts',(58.1000024265854,-4.56351680928159,25.7088785017885));
#7253=CARTESIAN_POINT('Ctrl Pts',(58.1000024265854,-12.9400663695712,22.4146400340441));
#7254=CARTESIAN_POINT('Ctrl Pts',(58.1000024265854,-18.9759447678742,17.605462615804));
#7255=CARTESIAN_POINT('Ctrl Pts',(58.1000024265854,-23.3131484812071,11.2309643464758));
#7256=CARTESIAN_POINT('Ctrl Pts',(58.1000024265854,-26.3712395611192,1.39808585601947));
#7257=CARTESIAN_POINT('Ctrl Pts',(58.1000024265854,-24.7843572520144,-9.10841329052855));
#7258=CARTESIAN_POINT('Ctrl Pts',(58.1000024265854,-18.9698058892659,-17.6032366064994));
#7259=CARTESIAN_POINT('Ctrl Pts',(58.1000024265854,-12.9431119186369,-22.4178983444412));
#7260=CARTESIAN_POINT('Ctrl Pts',(58.1000024265853,-5.76050665590931,-25.2279644925147));
#7261=CARTESIAN_POINT('Ctrl Pts',(58.1000024265854,4.50426658309875,-26.0207692060419));
#7262=CARTESIAN_POINT('Ctrl Pts',(58.1000024265854,15.6334530375707,-21.6527576889412));
#7263=CARTESIAN_POINT('Ctrl Pts',(58.1000024265854,23.7576198677921,-11.4339468021644));
#7264=CARTESIAN_POINT('Ctrl Pts',(58.1000024265854,25.4995308359827,-3.81455041897075));
#7265=CARTESIAN_POINT('Ctrl Pts',(58.1000024265854,25.4995308359827,7.66056040565432E-14));
#7266=CARTESIAN_POINT('Ctrl Pts',(58.1,25.5004302023323,2.38710372417893E-14));
#7267=CARTESIAN_POINT('Ctrl Pts',(58.1,25.5004302023323,3.81468495784946));
#7268=CARTESIAN_POINT('Ctrl Pts',(58.1,23.7611224475672,11.4418465836341));
#7269=CARTESIAN_POINT('Ctrl Pts',(58.1,16.4431730728752,20.6180326245795));
#7270=CARTESIAN_POINT('Ctrl Pts',(58.1,5.86849713807706,25.7112413848538));
#7271=CARTESIAN_POINT('Ctrl Pts',(58.1,-4.56367776414296,25.7097852518122));
#7272=CARTESIAN_POINT('Ctrl Pts',(58.1,-12.9405227646445,22.4154305965488));
#7273=CARTESIAN_POINT('Ctrl Pts',(58.1,-18.9766140478806,17.606083559018));
#7274=CARTESIAN_POINT('Ctrl Pts',(58.1,-23.3139707340307,11.2313604616617));
#7275=CARTESIAN_POINT('Ctrl Pts',(58.1000000000001,-26.3721696725628,1.39813516639225));
#7276=CARTESIAN_POINT('Ctrl Pts',(58.1,-24.78523139425,-9.10873454351383));
#7277=CARTESIAN_POINT('Ctrl Pts',(58.1000000000001,-18.9704749527546,-17.6038574712023));
#7278=CARTESIAN_POINT('Ctrl Pts',(58.1,-12.9435684211264,-22.4186890218663));
#7279=CARTESIAN_POINT('Ctrl Pts',(58.1,-5.7607098285038,-25.228854280741));
#7280=CARTESIAN_POINT('Ctrl Pts',(58.1,4.50442544820952,-26.021686956425));
#7281=CARTESIAN_POINT('Ctrl Pts',(58.1,15.6340044281696,-21.6535213799185));
#7282=CARTESIAN_POINT('Ctrl Pts',(58.1,23.7584577970848,-11.4343500765248));
#7283=CARTESIAN_POINT('Ctrl Pts',(58.1,25.5004302023316,-3.81468495784933));
#7284=CARTESIAN_POINT('Ctrl Pts',(58.1,25.5004302023316,7.6605795167492E-14));
#7285=CARTESIAN_POINT('Ctrl Pts',(58.1,25.5013295686812,2.38716421746933E-14));
#7286=CARTESIAN_POINT('Ctrl Pts',(58.1,25.5013295686812,3.81481949672803));
#7287=CARTESIAN_POINT('Ctrl Pts',(58.1,23.7619604708386,11.4422501223864));
#7288=CARTESIAN_POINT('Ctrl Pts',(58.1,16.4437530017789,20.6187597952419));
#7289=CARTESIAN_POINT('Ctrl Pts',(58.1,5.86870411218699,25.7121481862334));
#7290=CARTESIAN_POINT('Ctrl Pts',(58.1,-4.56383871900433,25.7106920018359));
#7291=CARTESIAN_POINT('Ctrl Pts',(58.1,-12.9409791597178,22.4162211590536));
#7292=CARTESIAN_POINT('Ctrl Pts',(58.1,-18.977283327887,17.606704502232));
#7293=CARTESIAN_POINT('Ctrl Pts',(58.1,-23.3147929868542,11.2317565768476));
#7294=CARTESIAN_POINT('Ctrl Pts',(58.1000000000001,-26.3730997840064,1.39818447676506));
#7295=CARTESIAN_POINT('Ctrl Pts',(58.1,-24.7861055364855,-9.10905579649912));
#7296=CARTESIAN_POINT('Ctrl Pts',(58.1000000000001,-18.9711440162433,-17.6044783359051));
#7297=CARTESIAN_POINT('Ctrl Pts',(58.1,-12.944024923616,-22.4194796992914));
#7298=CARTESIAN_POINT('Ctrl Pts',(58.1,-5.76091300109831,-25.2297440689673));
#7299=CARTESIAN_POINT('Ctrl Pts',(58.1,4.5045843133203,-26.0226047068082));
#7300=CARTESIAN_POINT('Ctrl Pts',(58.1,15.6345558187685,-21.6542850708958));
#7301=CARTESIAN_POINT('Ctrl Pts',(58.1,23.7592957263775,-11.4347533508852));
#7302=CARTESIAN_POINT('Ctrl Pts',(58.1,25.5013295686804,-3.8148194967279));
#7303=CARTESIAN_POINT('Ctrl Pts',(58.1,25.5013295686804,7.66059620291998E-14));
#7304=CARTESIAN_POINT('',(58.1,25.5013295686804,7.16093850883226E-14));
#7305=CARTESIAN_POINT('Origin',(58.6,25.5013295686812,2.16493489801906E-14));
#7306=CARTESIAN_POINT('Ctrl Pts',(58.1,25.5013295686797,7.54957705575713E-14));
#7307=CARTESIAN_POINT('Ctrl Pts',(58.1,25.5013295686797,-3.81481949672779));
#7308=CARTESIAN_POINT('Ctrl Pts',(58.1,24.6303126475283,-7.62478642380632));
#7309=CARTESIAN_POINT('Ctrl Pts',(58.1,22.9760932008113,-11.0626996453471));
#7310=CARTESIAN_POINT('Ctrl Pts',(58.1,21.3218737540942,-14.500612866888));
#7311=CARTESIAN_POINT('Ctrl Pts',(58.1,18.8844517818116,-17.5664723828911));
#7312=CARTESIAN_POINT('Ctrl Pts',(58.1,15.9016432968718,-19.9424377685946));
#7313=CARTESIAN_POINT('Ctrl Pts',(58.1,11.9245653169521,-23.1103916161994));
#7314=CARTESIAN_POINT('Ctrl Pts',(58.1,6.97791131453084,-25.0518670099382));
#7315=CARTESIAN_POINT('Ctrl Pts',(58.1,1.90719420891763,-25.4347385952375));
#7316=CARTESIAN_POINT('Ctrl Pts',(58.1,-0.628164343888988,-25.6261743878872));
#7317=CARTESIAN_POINT('Ctrl Pts',(58.1,-3.19453867249359,-25.427959228427));
#7318=CARTESIAN_POINT('Ctrl Pts',(58.1,-5.67491115721548,-24.8604742537509));
#7319=CARTESIAN_POINT('Ctrl Pts',(58.1,-8.15528364193736,-24.2929892790749));
#7320=CARTESIAN_POINT('Ctrl Pts',(58.1,-10.5496542827765,-23.3562344891829));
#7321=CARTESIAN_POINT('Ctrl Pts',(58.1,-12.7513594519673,-22.0853568670059));
#7322=CARTESIAN_POINT('Ctrl Pts',(58.1,-14.9530646211581,-20.8144792448289));
#7323=CARTESIAN_POINT('Ctrl Pts',(58.1,-16.9621043187005,-19.2094787903669));
#7324=CARTESIAN_POINT('Ctrl Pts',(58.1,-18.693494357502,-17.3450507457101));
#7325=CARTESIAN_POINT('Ctrl Pts',(58.1,-20.4248843963035,-15.4806227010533));
#7326=CARTESIAN_POINT('Ctrl Pts',(58.1,-21.878624776364,-13.3567670662019));
#7327=CARTESIAN_POINT('Ctrl Pts',(58.1,-22.9800345503645,-11.0652599535289));
#7328=CARTESIAN_POINT('Ctrl Pts',(58.1,-25.1828540983653,-6.48224572818298));
#7329=CARTESIAN_POINT('Ctrl Pts',(58.1,-25.9763512221258,-1.22862559155098));
#7330=CARTESIAN_POINT('Ctrl Pts',(58.1,-25.2214146643286,3.80043848735385));
#7331=CARTESIAN_POINT('Ctrl Pts',(58.1,-24.84394638543,6.31497052680626));
#7332=CARTESIAN_POINT('Ctrl Pts',(58.1,-24.0793696861419,8.77336355182689));
#7333=CARTESIAN_POINT('Ctrl Pts',(58.1,-22.9741630600034,11.0650513852346));
#7334=CARTESIAN_POINT('Ctrl Pts',(58.1,-21.8689564338649,13.3567392186423));
#7335=CARTESIAN_POINT('Ctrl Pts',(58.1,-20.4231198808759,15.481721860437));
#7336=CARTESIAN_POINT('Ctrl Pts',(58.1,-18.6941509096865,17.3457992908047));
#7337=CARTESIAN_POINT('Ctrl Pts',(58.1,-16.9651819384971,19.2098767211723));
#7338=CARTESIAN_POINT('Ctrl Pts',(58.1,-14.9530805491074,20.8130489401129));
#7339=CARTESIAN_POINT('Ctrl Pts',(58.1,-12.7502955057392,22.0852737414092));
#7340=CARTESIAN_POINT('Ctrl Pts',(58.1,-10.547510462371,23.3574985427055));
#7341=CARTESIAN_POINT('Ctrl Pts',(58.1,-8.15404176502431,24.2987759263576));
#7342=CARTESIAN_POINT('Ctrl Pts',(58.1,-5.67470626349718,24.8636879749886));
#7343=CARTESIAN_POINT('Ctrl Pts',(58.1,-1.95570301120648,25.7110560479351));
#7344=CARTESIAN_POINT('Ctrl Pts',(58.1,1.95650055049023,25.7116021170842));
#7345=CARTESIAN_POINT('Ctrl Pts',(58.1,5.6751104796039,24.8629770864935));
#7346=CARTESIAN_POINT('Ctrl Pts',(58.1,9.39372040871756,24.0143520559028));
#7347=CARTESIAN_POINT('Ctrl Pts',(58.1,12.9187367052482,22.3165559255723));
#7348=CARTESIAN_POINT('Ctrl Pts',(58.1,15.9009460983568,19.9382395815978));
#7349=CARTESIAN_POINT('Ctrl Pts',(58.1,18.8831554914654,17.5599232376234));
#7350=CARTESIAN_POINT('Ctrl Pts',(58.1,21.322557981152,14.5010866800049));
#7351=CARTESIAN_POINT('Ctrl Pts',(58.1,22.9771015004559,11.0648107447811));
#7352=CARTESIAN_POINT('Ctrl Pts',(58.1,24.6316450197599,7.62853480955721));
#7353=CARTESIAN_POINT('Ctrl Pts',(58.1,25.5013295686812,3.81481949672803));
#7354=CARTESIAN_POINT('Ctrl Pts',(58.1,25.5013295686812,2.38716421746933E-14));
#7355=CARTESIAN_POINT('Origin',(58.1,60.5,0.));
#7356=CARTESIAN_POINT('',(58.1,-7.3111413909097E-15,59.7));
#7357=CARTESIAN_POINT('Origin',(58.1,0.,0.));
#7358=CARTESIAN_POINT('Origin',(60.55,59.9249530663145,-3.));
#7359=CARTESIAN_POINT('',(60.6,59.9478721217627,-2.50052555931523));
#7360=CARTESIAN_POINT('',(60.6,59.9249530663145,-2.5));
#7361=CARTESIAN_POINT('Origin',(60.6,59.9249530663145,-3.));
#7362=CARTESIAN_POINT('',(62.4,59.9249530663145,-2.5));
#7363=CARTESIAN_POINT('',(60.55,59.9249530663145,-2.5));
#7364=CARTESIAN_POINT('',(62.4,60.4243276752005,-3.025));
#7365=CARTESIAN_POINT('Origin',(62.4,59.9249530663145,-3.));
#7366=CARTESIAN_POINT('',(60.1,60.4243276752005,-3.025));
#7367=CARTESIAN_POINT('',(60.55,60.4243276752005,-3.025));
#7368=CARTESIAN_POINT('Ctrl Pts',(60.6,59.9478721217627,-2.50052555931523));
#7369=CARTESIAN_POINT('Ctrl Pts',(60.6,59.9513712471188,-2.50068612138112));
#7370=CARTESIAN_POINT('Ctrl Pts',(60.5999631921872,59.9548737120599,-2.50088368385959));
#7371=CARTESIAN_POINT('Ctrl Pts',(60.5988534347359,60.0074936809125,-2.50440931235234));
#7372=CARTESIAN_POINT('Ctrl Pts',(60.5905898947881,60.0547893216016,-2.51485483908352));
#7373=CARTESIAN_POINT('Ctrl Pts',(60.5587918082573,60.1527949769169,-2.55124410360599));
#7374=CARTESIAN_POINT('Ctrl Pts',(60.5329987364422,60.2000785105811,-2.57930326175212));
#7375=CARTESIAN_POINT('Ctrl Pts',(60.4622024183735,60.292853998527,-2.65468544195021));
#7376=CARTESIAN_POINT('Ctrl Pts',(60.4115325491484,60.3362328533458,-2.70762122730265));
#7377=CARTESIAN_POINT('Ctrl Pts',(60.2769563903468,60.4089098807044,-2.8463207295033));
#7378=CARTESIAN_POINT('Ctrl Pts',(60.190541226799,60.428444844956,-2.93417456909241));
#7379=CARTESIAN_POINT('Ctrl Pts',(60.1015881345704,60.4244055071003,-3.02340716123007));
#7380=CARTESIAN_POINT('Ctrl Pts',(60.1007940667366,60.4243675436247,-3.02420362885069));
#7381=CARTESIAN_POINT('Ctrl Pts',(60.1,60.4243276752005,-3.025));
#7382=CARTESIAN_POINT('Ctrl Pts',(62.4,59.9249530663145,-2.5));
#7383=CARTESIAN_POINT('Ctrl Pts',(62.4261954145561,59.9249530663145,-2.5));
#7384=CARTESIAN_POINT('Ctrl Pts',(62.4783266322709,59.9031781113224,-2.5));
#7385=CARTESIAN_POINT('Ctrl Pts',(62.5,59.8510230365392,-2.5));
#7386=CARTESIAN_POINT('Ctrl Pts',(62.5,59.8248276219832,-2.5));
#7387=CARTESIAN_POINT('Ctrl Pts',(62.4,60.0600211649479,-2.5));
#7388=CARTESIAN_POINT('Ctrl Pts',(62.4616961972161,60.0600211649479,-2.5));
#7389=CARTESIAN_POINT('Ctrl Pts',(62.5841180518885,60.0076626751897,-2.49996163393935));
#7390=CARTESIAN_POINT('Ctrl Pts',(62.6320023421471,59.8852898118316,-2.49996440018845));
#7391=CARTESIAN_POINT('Ctrl Pts',(62.6308996938996,59.8248276219832,-2.5));
#7392=CARTESIAN_POINT('Ctrl Pts',(62.4,60.3287554028045,-2.61590736409158));
#7393=CARTESIAN_POINT('Ctrl Pts',(62.5319883255722,60.3287554028045,-2.61590736409158));
#7394=CARTESIAN_POINT('Ctrl Pts',(62.7941599982643,60.2152911717712,-2.61426659004369));
#7395=CARTESIAN_POINT('Ctrl Pts',(62.8947191636549,59.9532224176658,-2.61040576784208));
#7396=CARTESIAN_POINT('Ctrl Pts',(62.8915104141356,59.8248276219832,-2.60848958586446));
#7397=CARTESIAN_POINT('Ctrl Pts',(62.4,60.4310810801322,-2.89010084214397));
#7398=CARTESIAN_POINT('Ctrl Pts',(62.5592604005367,60.4310810801322,-2.89010084214397));
#7399=CARTESIAN_POINT('Ctrl Pts',(62.8753088977623,60.2975536797591,-2.8854985007134));
#7400=CARTESIAN_POINT('Ctrl Pts',(63.0017539553834,59.9819463835178,-2.87456299295786));
#7401=CARTESIAN_POINT('Ctrl Pts',(63.,59.8248276219832,-2.86910030610043));
#7402=CARTESIAN_POINT('Ctrl Pts',(62.4,60.4243276752005,-3.02500000000001));
#7403=CARTESIAN_POINT('Ctrl Pts',(62.5571724873364,60.4243276752005,-3.02500000000001));
#7404=CARTESIAN_POINT('Ctrl Pts',(62.8699597936253,60.2939494729186,-3.01957486519097));
#7405=CARTESIAN_POINT('Ctrl Pts',(63.,59.9816715724272,-3.00655155431689));
#7406=CARTESIAN_POINT('Ctrl Pts',(63.,59.8248276219832,-3.));
#7407=CARTESIAN_POINT('',(62.5,59.8248276219832,-2.5));
#7408=CARTESIAN_POINT('',(63.,59.8248276219832,-3.));
#7409=CARTESIAN_POINT('Origin',(62.5,59.8248276219832,-3.));
#7410=CARTESIAN_POINT('Ctrl Pts',(63.,59.8248276219832,-3.));
#7411=CARTESIAN_POINT('Ctrl Pts',(63.,59.9816715724272,-3.00655155431689));
#7412=CARTESIAN_POINT('Ctrl Pts',(62.8699597936253,60.2939494729186,-3.01957486519097));
#7413=CARTESIAN_POINT('Ctrl Pts',(62.5571724873364,60.4243276752005,-3.02500000000001));
#7414=CARTESIAN_POINT('Ctrl Pts',(62.4,60.4243276752005,-3.02500000000001));
#7415=CARTESIAN_POINT('Ctrl Pts',(62.4,59.9249530663145,-2.5));
#7416=CARTESIAN_POINT('Ctrl Pts',(62.4261954145561,59.9249530663145,-2.5));
#7417=CARTESIAN_POINT('Ctrl Pts',(62.4783266322709,59.9031781113224,-2.5));
#7418=CARTESIAN_POINT('Ctrl Pts',(62.5,59.8510230365392,-2.5));
#7419=CARTESIAN_POINT('Ctrl Pts',(62.5,59.8248276219832,-2.5));
#7420=CARTESIAN_POINT('Origin',(62.5,58.25,-3.));
#7421=CARTESIAN_POINT('',(62.5,58.0224956374681,-2.5));
#7422=CARTESIAN_POINT('',(63.,58.0224956374681,-3.));
#7423=CARTESIAN_POINT('Origin',(62.5,58.0224956374681,-3.));
#7424=CARTESIAN_POINT('',(63.,58.25,-3.));
#7425=CARTESIAN_POINT('',(62.5,58.25,-2.5));
#7426=CARTESIAN_POINT('Ctrl Pts',(62.5,58.0224956374681,-2.5));
#7427=CARTESIAN_POINT('Ctrl Pts',(62.5,57.9962991377946,-2.5));
#7428=CARTESIAN_POINT('Ctrl Pts',(62.478326631158,57.9441387853006,-2.5));
#7429=CARTESIAN_POINT('Ctrl Pts',(62.4261964996734,57.9223618302983,-2.5));
#7430=CARTESIAN_POINT('Ctrl Pts',(62.4,57.9223618302983,-2.5));
#7431=CARTESIAN_POINT('Ctrl Pts',(62.6308996938996,58.0224956374681,-2.5));
#7432=CARTESIAN_POINT('Ctrl Pts',(62.6297629272861,57.9620363652066,-2.50003670134814));
#7433=CARTESIAN_POINT('Ctrl Pts',(62.5778246198969,57.8438878491714,-2.50003956584365));
#7434=CARTESIAN_POINT('Ctrl Pts',(62.4594554053708,57.795774405517,-2.5));
#7435=CARTESIAN_POINT('Ctrl Pts',(62.4,57.795774405517,-2.5));
#7436=CARTESIAN_POINT('Ctrl Pts',(62.8915113750724,58.022495637468,-2.60848862492762));
#7437=CARTESIAN_POINT('Ctrl Pts',(62.8882033397738,57.8941116945847,-2.60651315205814));
#7438=CARTESIAN_POINT('Ctrl Pts',(62.7758463976871,57.6445251096574,-2.60266612956143));
#7439=CARTESIAN_POINT('Ctrl Pts',(62.5254658026268,57.5435955938278,-2.60110845458278));
#7440=CARTESIAN_POINT('Ctrl Pts',(62.4,57.5435955938278,-2.60110845458278));
#7441=CARTESIAN_POINT('Ctrl Pts',(63.,58.0224956374681,-2.86910030610043));
#7442=CARTESIAN_POINT('Ctrl Pts',(62.998191773373,57.865391083981,-2.86346859167697));
#7443=CARTESIAN_POINT('Ctrl Pts',(62.8652984129375,57.5564336213585,-2.85232926567146));
#7444=CARTESIAN_POINT('Ctrl Pts',(62.5556992082037,57.4295787502844,-2.84771995480427));
#7445=CARTESIAN_POINT('Ctrl Pts',(62.4,57.4295787502844,-2.84771995480427));
#7446=CARTESIAN_POINT('Ctrl Pts',(63.,58.0224956374681,-3.00000000000001));
#7447=CARTESIAN_POINT('Ctrl Pts',(63.,57.8656658629709,-2.99324572615905));
#7448=CARTESIAN_POINT('Ctrl Pts',(62.8699597869483,57.5534008162154,-2.97977498708946));
#7449=CARTESIAN_POINT('Ctrl Pts',(62.5571789980404,57.4230311248647,-2.97413793103448));
#7450=CARTESIAN_POINT('Ctrl Pts',(62.4,57.4230311248647,-2.97413793103448));
#7451=CARTESIAN_POINT('',(62.4,57.9223618302983,-2.5));
#7452=CARTESIAN_POINT('',(62.4,57.4230311248647,-2.97413793103448));
#7453=CARTESIAN_POINT('Origin',(62.4,57.9223618302983,-3.));
#7454=CARTESIAN_POINT('Ctrl Pts',(62.4,57.4230311248647,-2.97413793103448));
#7455=CARTESIAN_POINT('Ctrl Pts',(62.5571789980404,57.4230311248647,-2.97413793103448));
#7456=CARTESIAN_POINT('Ctrl Pts',(62.8699597869483,57.5534008162154,-2.97977498708946));
#7457=CARTESIAN_POINT('Ctrl Pts',(63.,57.8656658629709,-2.99324572615905));
#7458=CARTESIAN_POINT('Ctrl Pts',(63.,58.0224956374681,-3.00000000000001));
#7459=CARTESIAN_POINT('Ctrl Pts',(62.5,58.0224956374681,-2.5));
#7460=CARTESIAN_POINT('Ctrl Pts',(62.5,57.9962991377946,-2.5));
#7461=CARTESIAN_POINT('Ctrl Pts',(62.478326631158,57.9441387853006,-2.5));
#7462=CARTESIAN_POINT('Ctrl Pts',(62.4261964996734,57.9223618302983,-2.5));
#7463=CARTESIAN_POINT('Ctrl Pts',(62.4,57.9223618302983,-2.5));
#7464=CARTESIAN_POINT('Origin',(61.55,57.9223618302983,-3.));
#7465=CARTESIAN_POINT('',(60.5994374367416,57.9223618302896,-2.5));
#7466=CARTESIAN_POINT('Ctrl Pts',(60.1,57.4230311248647,-2.97413793103448));
#7467=CARTESIAN_POINT('Ctrl Pts',(60.1008135540983,57.4230730234755,-2.97332897553566));
#7468=CARTESIAN_POINT('Ctrl Pts',(60.1016271094375,57.4231168880088,-2.97252012062025));
#7469=CARTESIAN_POINT('Ctrl Pts',(60.1591133854327,57.4263552929666,-2.91537316521117));
#7470=CARTESIAN_POINT('Ctrl Pts',(60.2161905779351,57.439110580143,-2.8591262187641));
#7471=CARTESIAN_POINT('Ctrl Pts',(60.3268065827896,57.4846962962046,-2.75111321481816));
#7472=CARTESIAN_POINT('Ctrl Pts',(60.3812501918161,57.5182917420481,-2.69848124864027));
#7473=CARTESIAN_POINT('Ctrl Pts',(60.4681999917132,57.5985821334825,-2.61563853552119));
#7474=CARTESIAN_POINT('Ctrl Pts',(60.5033113035832,57.6412749470976,-2.58265302130672));
#7475=CARTESIAN_POINT('Ctrl Pts',(60.554272023061,57.7307439456096,-2.53604375043298));
#7476=CARTESIAN_POINT('Ctrl Pts',(60.5724543137632,57.7744341680491,-2.51995587221209));
#7477=CARTESIAN_POINT('Ctrl Pts',(60.5927186872872,57.8544686959718,-2.50350008622553));
#7478=CARTESIAN_POINT('Ctrl Pts',(60.5978171938089,57.8882030869101,-2.5000000000006));
#7479=CARTESIAN_POINT('Ctrl Pts',(60.599437436742,57.9223618302896,-2.5));
#7480=CARTESIAN_POINT('',(61.55,57.4230311248647,-2.97413793103448));
#7481=CARTESIAN_POINT('',(61.55,57.9223618302983,-2.5));
#7482=CARTESIAN_POINT('Origin',(62.3,59.,-2.5));
#7483=CARTESIAN_POINT('',(60.6,57.9460956406901,-2.5));
#7484=CARTESIAN_POINT('',(60.6,61.5,-2.5));
#7485=CARTESIAN_POINT('Ctrl Pts',(60.6,57.9460956406901,-2.5));
#7486=CARTESIAN_POINT('Ctrl Pts',(60.6,57.9383411366579,-2.5));
#7487=CARTESIAN_POINT('Ctrl Pts',(60.5998192566414,57.9304115416576,-2.5));
#7488=CARTESIAN_POINT('Ctrl Pts',(60.599437436742,57.9223618302896,-2.5));
#7489=CARTESIAN_POINT('Origin',(61.55,57.9223618302983,3.));
#7490=CARTESIAN_POINT('',(60.5994374367416,57.9223618302896,2.5));
#7491=CARTESIAN_POINT('Ctrl Pts',(60.599437436742,57.9223618302896,2.5));
#7492=CARTESIAN_POINT('Ctrl Pts',(60.5978171938089,57.8882030869104,2.5000000000006));
#7493=CARTESIAN_POINT('Ctrl Pts',(60.5927186872873,57.8544686959723,2.50350008622548));
#7494=CARTESIAN_POINT('Ctrl Pts',(60.5724543137635,57.7744341680499,2.51995587221184));
#7495=CARTESIAN_POINT('Ctrl Pts',(60.5542720230614,57.7307439456104,2.53604375043265));
#7496=CARTESIAN_POINT('Ctrl Pts',(60.5033113035838,57.6412749470984,2.58265302130619));
#7497=CARTESIAN_POINT('Ctrl Pts',(60.468199991714,57.5985821334833,2.61563853552051));
#7498=CARTESIAN_POINT('Ctrl Pts',(60.3812501918168,57.5182917420486,2.69848124863954));
#7499=CARTESIAN_POINT('Ctrl Pts',(60.3268065827902,57.4846962962049,2.75111321481755));
#7500=CARTESIAN_POINT('Ctrl Pts',(60.2161905779354,57.439110580143,2.85912621876381));
#7501=CARTESIAN_POINT('Ctrl Pts',(60.1591133854132,57.4263552929677,2.91537316519053));
#7502=CARTESIAN_POINT('Ctrl Pts',(60.1016271094397,57.4231168880088,2.97252012062051));
#7503=CARTESIAN_POINT('Ctrl Pts',(60.1008135540976,57.4230730234755,2.9733289755364));
#7504=CARTESIAN_POINT('Ctrl Pts',(60.1,57.4230311248647,2.97413793103449));
#7505=CARTESIAN_POINT('',(62.4,57.9223618302983,2.5));
#7506=CARTESIAN_POINT('',(61.55,57.9223618302983,2.5));
#7507=CARTESIAN_POINT('',(62.4,57.4230311248647,2.97413793103448));
#7508=CARTESIAN_POINT('Origin',(62.4,57.9223618302983,3.));
#7509=CARTESIAN_POINT('',(61.55,57.4230311248647,2.97413793103448));
#7510=CARTESIAN_POINT('Ctrl Pts',(62.4,57.9223618302983,2.5));
#7511=CARTESIAN_POINT('Ctrl Pts',(62.4261965009078,57.9223618302983,2.5));
#7512=CARTESIAN_POINT('Ctrl Pts',(62.478328938404,57.9441410931384,2.5));
#7513=CARTESIAN_POINT('Ctrl Pts',(62.5,57.9962991365602,2.5));
#7514=CARTESIAN_POINT('Ctrl Pts',(62.5,58.0224956374681,2.5));
#7515=CARTESIAN_POINT('Ctrl Pts',(62.4,57.795774405517,2.5));
#7516=CARTESIAN_POINT('Ctrl Pts',(62.4594554081724,57.795774405517,2.5));
#7517=CARTESIAN_POINT('Ctrl Pts',(62.5778299501554,57.8438930222843,2.50003956285446));
#7518=CARTESIAN_POINT('Ctrl Pts',(62.6297629272325,57.9620363623577,2.50003670134987));
#7519=CARTESIAN_POINT('Ctrl Pts',(62.6308996938996,58.0224956374681,2.5));
#7520=CARTESIAN_POINT('Ctrl Pts',(62.4,57.5435955938278,2.60110845458278));
#7521=CARTESIAN_POINT('Ctrl Pts',(62.525465808539,57.5435955938278,2.60110845458278));
#7522=CARTESIAN_POINT('Ctrl Pts',(62.7758577213737,57.6445359736439,2.60266629871633));
#7523=CARTESIAN_POINT('Ctrl Pts',(62.8882033396179,57.894111688535,2.60651315196505));
#7524=CARTESIAN_POINT('Ctrl Pts',(62.8915113750724,58.022495637468,2.60848862492761));
#7525=CARTESIAN_POINT('Ctrl Pts',(62.4,57.4295787502844,2.84771995480428));
#7526=CARTESIAN_POINT('Ctrl Pts',(62.5556992155405,57.4295787502844,2.84771995480428));
#7527=CARTESIAN_POINT('Ctrl Pts',(62.8653122771054,57.5564472161643,2.85232975672316));
#7528=CARTESIAN_POINT('Ctrl Pts',(62.9981917732878,57.865391076578,2.86346859141159));
#7529=CARTESIAN_POINT('Ctrl Pts',(63.,58.0224956374681,2.86910030610042));
#7530=CARTESIAN_POINT('Ctrl Pts',(62.4,57.4230311248647,2.97413793103449));
#7531=CARTESIAN_POINT('Ctrl Pts',(62.5571790054469,57.4230311248647,2.97413793103449));
#7532=CARTESIAN_POINT('Ctrl Pts',(62.8699736304242,57.5534146323498,2.9797755837571));
#7533=CARTESIAN_POINT('Ctrl Pts',(63.,57.8656658555809,2.99324572584077));
#7534=CARTESIAN_POINT('Ctrl Pts',(63.,58.0224956374681,3.));
#7535=CARTESIAN_POINT('',(62.5,58.0224956374681,2.5));
#7536=CARTESIAN_POINT('',(63.,58.0224956374681,3.));
#7537=CARTESIAN_POINT('Origin',(62.5,58.0224956374681,3.));
#7538=CARTESIAN_POINT('Ctrl Pts',(63.,58.0224956374681,3.));
#7539=CARTESIAN_POINT('Ctrl Pts',(63.,57.8656658555809,2.99324572584077));
#7540=CARTESIAN_POINT('Ctrl Pts',(62.8699736304242,57.5534146323498,2.9797755837571));
#7541=CARTESIAN_POINT('Ctrl Pts',(62.5571790054469,57.4230311248647,2.97413793103449));
#7542=CARTESIAN_POINT('Ctrl Pts',(62.4,57.4230311248647,2.97413793103449));
#7543=CARTESIAN_POINT('Ctrl Pts',(62.4,57.9223618302983,2.5));
#7544=CARTESIAN_POINT('Ctrl Pts',(62.4261965009078,57.9223618302983,2.5));
#7545=CARTESIAN_POINT('Ctrl Pts',(62.478328938404,57.9441410931384,2.5));
#7546=CARTESIAN_POINT('Ctrl Pts',(62.5,57.9962991365602,2.5));
#7547=CARTESIAN_POINT('Ctrl Pts',(62.5,58.0224956374681,2.5));
#7548=CARTESIAN_POINT('Origin',(62.5,58.25,3.));
#7549=CARTESIAN_POINT('',(62.5,59.8248276219832,2.5));
#7550=CARTESIAN_POINT('',(63.,59.8248276219832,3.));
#7551=CARTESIAN_POINT('Origin',(62.5,59.8248276219832,3.));
#7552=CARTESIAN_POINT('',(63.,58.25,3.));
#7553=CARTESIAN_POINT('',(62.5,58.25,2.5));
#7554=CARTESIAN_POINT('Ctrl Pts',(62.5,59.8248276219832,2.5));
#7555=CARTESIAN_POINT('Ctrl Pts',(62.5,59.8510230353731,2.5));
#7556=CARTESIAN_POINT('Ctrl Pts',(62.4783243250786,59.9031804190904,2.5));
#7557=CARTESIAN_POINT('Ctrl Pts',(62.4261954133899,59.9249530663145,2.5));
#7558=CARTESIAN_POINT('Ctrl Pts',(62.4,59.9249530663145,2.5));
#7559=CARTESIAN_POINT('Ctrl Pts',(62.6308996938996,59.8248276219832,2.5));
#7560=CARTESIAN_POINT('Ctrl Pts',(62.632002342098,59.88528980914,2.49996440019004));
#7561=CARTESIAN_POINT('Ctrl Pts',(62.5841127217071,60.0076681632058,2.49996163056113));
#7562=CARTESIAN_POINT('Ctrl Pts',(62.4616961944695,60.0600211649479,2.5));
#7563=CARTESIAN_POINT('Ctrl Pts',(62.4,60.0600211649479,2.5));
#7564=CARTESIAN_POINT('Ctrl Pts',(62.8915104141354,59.8248276219832,2.6084895858646));
#7565=CARTESIAN_POINT('Ctrl Pts',(62.8947191635119,59.9532224119501,2.61040576775692));
#7566=CARTESIAN_POINT('Ctrl Pts',(62.7941486746792,60.2153029522765,2.61426676371213));
#7567=CARTESIAN_POINT('Ctrl Pts',(62.5319883196965,60.3287554028044,2.61590736409173));
#7568=CARTESIAN_POINT('Ctrl Pts',(62.4,60.3287554028044,2.61590736409173));
#7569=CARTESIAN_POINT('Ctrl Pts',(63.,59.8248276219832,2.86910030610042));
#7570=CARTESIAN_POINT('Ctrl Pts',(63.0017539553053,59.9819463765234,2.87456299271468));
#7571=CARTESIAN_POINT('Ctrl Pts',(62.8752950337675,60.2975677764337,2.88549898701103));
#7572=CARTESIAN_POINT('Ctrl Pts',(62.5592603934469,60.4310810801322,2.89010084214396));
#7573=CARTESIAN_POINT('Ctrl Pts',(62.4,60.4310810801322,2.89010084214396));
#7574=CARTESIAN_POINT('Ctrl Pts',(63.,59.8248276219832,3.));
#7575=CARTESIAN_POINT('Ctrl Pts',(63.,59.981671565445,3.00655155402523));
#7576=CARTESIAN_POINT('Ctrl Pts',(62.8699459504713,60.2939632906984,3.01957544083796));
#7577=CARTESIAN_POINT('Ctrl Pts',(62.5571724803396,60.4243276752005,3.025));
#7578=CARTESIAN_POINT('Ctrl Pts',(62.4,60.4243276752005,3.025));
#7579=CARTESIAN_POINT('',(62.4,59.9249530663145,2.5));
#7580=CARTESIAN_POINT('',(62.4,60.4243276752005,3.025));
#7581=CARTESIAN_POINT('Origin',(62.4,59.9249530663145,3.));
#7582=CARTESIAN_POINT('Ctrl Pts',(62.4,60.4243276752005,3.025));
#7583=CARTESIAN_POINT('Ctrl Pts',(62.5571724803396,60.4243276752005,3.025));
#7584=CARTESIAN_POINT('Ctrl Pts',(62.8699459504713,60.2939632906984,3.01957544083796));
#7585=CARTESIAN_POINT('Ctrl Pts',(63.,59.981671565445,3.00655155402523));
#7586=CARTESIAN_POINT('Ctrl Pts',(63.,59.8248276219832,3.));
#7587=CARTESIAN_POINT('Ctrl Pts',(62.5,59.8248276219832,2.5));
#7588=CARTESIAN_POINT('Ctrl Pts',(62.5,59.8510230353731,2.5));
#7589=CARTESIAN_POINT('Ctrl Pts',(62.4783243250786,59.9031804190904,2.5));
#7590=CARTESIAN_POINT('Ctrl Pts',(62.4261954133899,59.9249530663145,2.5));
#7591=CARTESIAN_POINT('Ctrl Pts',(62.4,59.9249530663145,2.5));
#7592=CARTESIAN_POINT('Origin',(60.55,59.9249530663145,3.));
#7593=CARTESIAN_POINT('',(60.1,60.4243276752005,3.025));
#7594=CARTESIAN_POINT('',(60.6,59.9478721217627,2.50052555931523));
#7595=CARTESIAN_POINT('Ctrl Pts',(60.1,60.4243276752005,3.02500000000001));
#7596=CARTESIAN_POINT('Ctrl Pts',(60.1007940667368,60.4243675436247,3.02420362885053));
#7597=CARTESIAN_POINT('Ctrl Pts',(60.1015881345702,60.4244055071002,3.02340716123028));
#7598=CARTESIAN_POINT('Ctrl Pts',(60.1905412267977,60.4284448449559,2.93417456909374));
#7599=CARTESIAN_POINT('Ctrl Pts',(60.2769563903458,60.408909880705,2.84632072950434));
#7600=CARTESIAN_POINT('Ctrl Pts',(60.4115325491487,60.3362328533456,2.70762122730233));
#7601=CARTESIAN_POINT('Ctrl Pts',(60.4622024183737,60.2928539985268,2.65468544195));
#7602=CARTESIAN_POINT('Ctrl Pts',(60.5329987364422,60.2000785105811,2.5793032617521));
#7603=CARTESIAN_POINT('Ctrl Pts',(60.5587918082574,60.1527949769168,2.55124410360597));
#7604=CARTESIAN_POINT('Ctrl Pts',(60.5905898947881,60.0547893216016,2.5148548390835));
#7605=CARTESIAN_POINT('Ctrl Pts',(60.5988534347359,60.0074936809124,2.50440931235233));
#7606=CARTESIAN_POINT('Ctrl Pts',(60.5999631921872,59.9548737120598,2.50088368385959));
#7607=CARTESIAN_POINT('Ctrl Pts',(60.6,59.9513712471188,2.50068612138112));
#7608=CARTESIAN_POINT('Ctrl Pts',(60.6,59.9478721217627,2.50052555931523));
#7609=CARTESIAN_POINT('',(60.55,60.4243276752005,3.025));
#7610=CARTESIAN_POINT('',(60.6,59.9249530663145,2.5));
#7611=CARTESIAN_POINT('',(60.55,59.9249530663145,2.5));
#7612=CARTESIAN_POINT('Origin',(60.6,59.9249530663145,3.));
#7613=CARTESIAN_POINT('Origin',(62.3,59.,2.5));
#7614=CARTESIAN_POINT('',(60.6,57.9460956406901,2.5));
#7615=CARTESIAN_POINT('Ctrl Pts',(60.599437436742,57.9223618302896,2.5));
#7616=CARTESIAN_POINT('Ctrl Pts',(60.5998192566414,57.9304115416576,2.5));
#7617=CARTESIAN_POINT('Ctrl Pts',(60.6,57.9383411366579,2.5));
#7618=CARTESIAN_POINT('Ctrl Pts',(60.6,57.9460956406901,2.5));
#7619=CARTESIAN_POINT('',(60.6,61.5,2.5));
#7620=CARTESIAN_POINT('Origin',(60.1,0.,0.));
#7621=CARTESIAN_POINT('Origin',(60.6,0.,0.));
#7622=CARTESIAN_POINT('Origin',(60.1,0.,0.));
#7623=CARTESIAN_POINT('Origin',(60.6,61.5,0.));
#7624=CARTESIAN_POINT('Origin',(60.6,0.,0.));
#7625=CARTESIAN_POINT('Origin',(60.1,0.,0.));
#7626=CARTESIAN_POINT('Origin',(61.55,0.,0.));
#7627=CARTESIAN_POINT('Origin',(62.4,0.,0.));
#7628=CARTESIAN_POINT('Origin',(62.4,0.,0.));
#7629=CARTESIAN_POINT('Origin',(63.,0.,0.));
#7630=CARTESIAN_POINT('Origin',(63.,57.5,0.));
#7631=CARTESIAN_POINT('Origin',(63.,0.,0.));
#7632=CARTESIAN_POINT('Origin',(60.55,0.,0.));
#7633=CARTESIAN_POINT('',(62.4,-60.5,-7.40911313484149E-15));
#7634=CARTESIAN_POINT('Origin',(62.4,0.,0.));
#7635=CARTESIAN_POINT('',(58.9,-60.5,-7.40911313484149E-15));
#7636=CARTESIAN_POINT('',(60.55,-60.5,-7.40911313484149E-15));
#7637=CARTESIAN_POINT('',(58.9,-7.40911313484149E-15,60.5));
#7638=CARTESIAN_POINT('Origin',(58.9,0.,0.));
#7639=CARTESIAN_POINT('Origin',(58.9,0.,0.));
#7640=CARTESIAN_POINT('Origin',(62.4,0.,0.));
#7641=CARTESIAN_POINT('Origin',(62.4,0.,0.));
#7642=CARTESIAN_POINT('Origin',(58.9,0.,0.));
#7643=CARTESIAN_POINT('Origin',(58.9,-7.3111413909097E-15,59.7));
#12791=UNCERTAINTY_MEASURE_WITH_UNIT(LENGTH_MEASURE(0.01),#12814,
'DISTANCE_ACCURACY_VALUE',
'Maximum model space distance between geometric entities at asserted c
onnectivities');
#12801=UNCERTAINTY_MEASURE_WITH_UNIT(LENGTH_MEASURE(0.01),#12814,
'DISTANCE_ACCURACY_VALUE',
'Maximum model space distance between geometric entities at asserted c
onnectivities');
#12803=(
GEOMETRIC_REPRESENTATION_CONTEXT(3)
GLOBAL_UNCERTAINTY_ASSIGNED_CONTEXT((#12791))
GLOBAL_UNIT_ASSIGNED_CONTEXT((#12814,#12816,#12817))
REPRESENTATION_CONTEXT('','3D')
);
#12813=(
GEOMETRIC_REPRESENTATION_CONTEXT(3)
GLOBAL_UNCERTAINTY_ASSIGNED_CONTEXT((#12801))
GLOBAL_UNIT_ASSIGNED_CONTEXT((#12814,#12816,#12817))
REPRESENTATION_CONTEXT('','3D')
);
#12814=(
LENGTH_UNIT()
NAMED_UNIT(*)
SI_UNIT(.MILLI.,.METRE.)
);
#12816=(
NAMED_UNIT(*)
PLANE_ANGLE_UNIT()
SI_UNIT($,.RADIAN.)
);
#12817=(
NAMED_UNIT(*)
SI_UNIT($,.STERADIAN.)
SOLID_ANGLE_UNIT()
);
#12819=SHAPE_DEFINITION_REPRESENTATION(#12830,#12854);
#12830=PRODUCT_DEFINITION_SHAPE('',$,#12866);
#12854=SHAPE_REPRESENTATION('',(#4506),#12803);
#12864=PRODUCT_DEFINITION_CONTEXT('part definition',#12899,'design');
#12866=PRODUCT_DEFINITION('2026-10-11-12-17-34-921',
'01_Upper_Fixed_Sheave_Flange',#12877,#12864);
#12877=PRODUCT_DEFINITION_FORMATION('',$,#12902);
#12899=APPLICATION_CONTEXT(
'Core Data for Automotive Mechanical Design Process');
#12900=PRODUCT_CONTEXT('part definition',#12899,'mechanical');
#12902=PRODUCT('2026-10-11-12-17-34-921','01_Upper_Fixed_Sheave_Flange',
$,(#12900));
#12954=COLOUR_RGB('Light Blue',0.38,0.62,0.78);
#12955=FILL_AREA_STYLE_COLOUR('',#12954);
#12956=FILL_AREA_STYLE('',(#12955));
#12957=SURFACE_STYLE_FILL_AREA(#12956);
#12958=SURFACE_SIDE_STYLE('',(#12957));
#12959=SURFACE_STYLE_USAGE(.BOTH.,#12958);
#12960=PRESENTATION_STYLE_ASSIGNMENT((#12959));
ENDSEC;
END-ISO-10303-21;
